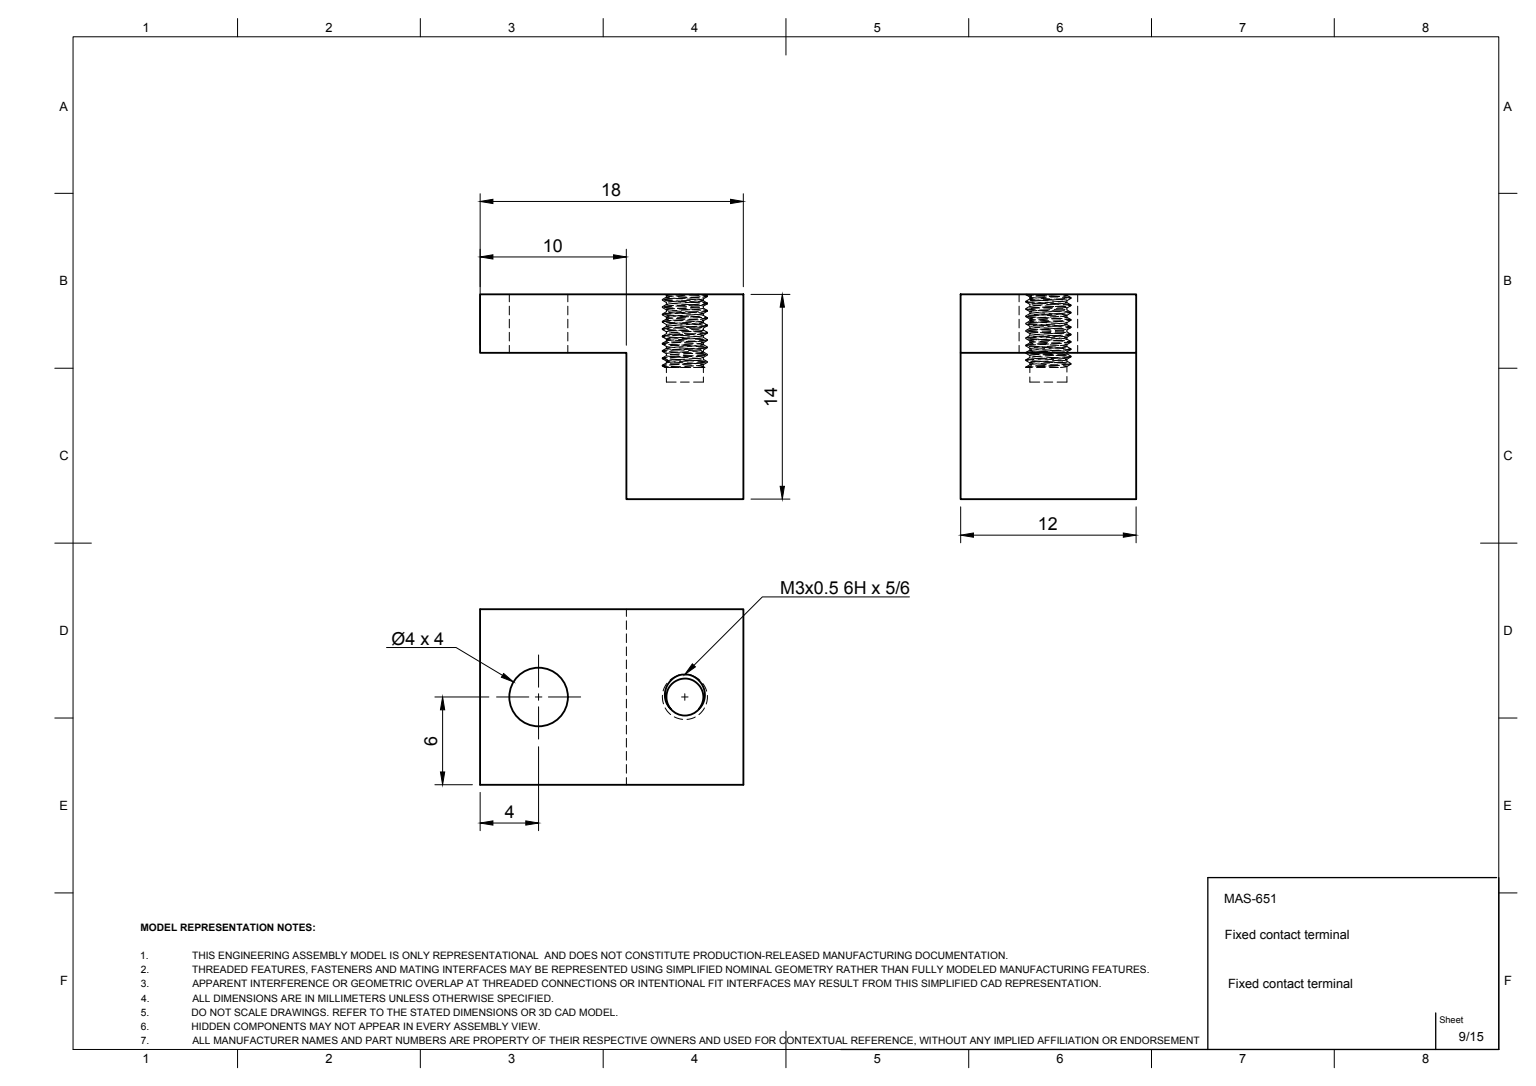
ISO-10303-21;
HEADER;
/* Generated by software containing ST-Developer
 * from STEP Tools, Inc. (www.steptools.com) 
 */

FILE_DESCRIPTION(
/* description */ ('Independent direct-acting normally-closed roller-plunger limit-switch
 CAD. Removable cover, insulated terminal supports, captured bus/conta
ct bridge, native Coil return spring, integral lower travel stop, reus
able instanced hardware and free roller. Manual geometric contact open
ing4mm; no snap-action/contact-force, electrical/current/voltage, envi
ronmental seal, safety-switch, wear, load or life certification. Exter
nal wiring and anchors omitted; fits and application engineering requi
red.'),
/* implementation_level */ '2;1');

FILE_NAME(
/* name */ 'Fixed contact terminal.step',
/* time_stamp */ '2026-11-08T07:32:43-08:00',
/* author */ (''),
/* organization */ (''),
/* preprocessor_version */ 'ST-DEVELOPER v20.2',
/* originating_system */ 'Autodesk Translation Framework v15.17.0.0',
/* authorisation */ '');

FILE_SCHEMA (('AUTOMOTIVE_DESIGN { 1 0 10303 214 3 1 1 }'));
ENDSEC;

DATA;
#10=MECHANICAL_DESIGN_GEOMETRIC_PRESENTATION_REPRESENTATION('',(#183),#36482);
#149=SHAPE_REPRESENTATION_RELATIONSHIP('SRR','None',#36562,#166);
#166=ADVANCED_BREP_SHAPE_REPRESENTATION('',(#200),#36472);
#183=STYLED_ITEM('',(#36653),#200);
#200=MANIFOLD_SOLID_BREP('Body1',#9774);
#226=B_SPLINE_SURFACE_WITH_KNOTS('',3,3,((#28474,#28475,#28476,#28477,#28478,
#28479,#28480,#28481,#28482,#28483,#28484,#28485,#28486,#28487,#28488,#28489,
#28490,#28491,#28492,#28493,#28494,#28495,#28496,#28497,#28498,#28499,#28500,
#28501,#28502,#28503,#28504,#28505,#28506,#28507,#28508,#28509,#28510,#28511,
#28512,#28513,#28514,#28515,#28516,#28517,#28518,#28519,#28520,#28521,#28522,
#28523,#28524,#28525,#28526,#28527,#28528,#28529,#28530,#28531,#28532,#28533,
#28534,#28535,#28536,#28537,#28538,#28539,#28540,#28541),(#28542,#28543,
#28544,#28545,#28546,#28547,#28548,#28549,#28550,#28551,#28552,#28553,#28554,
#28555,#28556,#28557,#28558,#28559,#28560,#28561,#28562,#28563,#28564,#28565,
#28566,#28567,#28568,#28569,#28570,#28571,#28572,#28573,#28574,#28575,#28576,
#28577,#28578,#28579,#28580,#28581,#28582,#28583,#28584,#28585,#28586,#28587,
#28588,#28589,#28590,#28591,#28592,#28593,#28594,#28595,#28596,#28597,#28598,
#28599,#28600,#28601,#28602,#28603,#28604,#28605,#28606,#28607,#28608,#28609),
(#28610,#28611,#28612,#28613,#28614,#28615,#28616,#28617,#28618,#28619,
#28620,#28621,#28622,#28623,#28624,#28625,#28626,#28627,#28628,#28629,#28630,
#28631,#28632,#28633,#28634,#28635,#28636,#28637,#28638,#28639,#28640,#28641,
#28642,#28643,#28644,#28645,#28646,#28647,#28648,#28649,#28650,#28651,#28652,
#28653,#28654,#28655,#28656,#28657,#28658,#28659,#28660,#28661,#28662,#28663,
#28664,#28665,#28666,#28667,#28668,#28669,#28670,#28671,#28672,#28673,#28674,
#28675,#28676,#28677),(#28678,#28679,#28680,#28681,#28682,#28683,#28684,
#28685,#28686,#28687,#28688,#28689,#28690,#28691,#28692,#28693,#28694,#28695,
#28696,#28697,#28698,#28699,#28700,#28701,#28702,#28703,#28704,#28705,#28706,
#28707,#28708,#28709,#28710,#28711,#28712,#28713,#28714,#28715,#28716,#28717,
#28718,#28719,#28720,#28721,#28722,#28723,#28724,#28725,#28726,#28727,#28728,
#28729,#28730,#28731,#28732,#28733,#28734,#28735,#28736,#28737,#28738,#28739,
#28740,#28741,#28742,#28743,#28744,#28745)),.UNSPECIFIED.,.F.,.F.,.F.,(4,
4),(4,1,1,1,1,1,1,1,1,1,1,1,1,1,1,1,1,1,1,1,1,1,1,1,1,1,1,1,1,1,1,1,1,1,
1,1,1,1,1,1,1,1,1,1,1,1,1,1,1,1,1,1,1,1,1,1,1,1,1,1,1,1,1,1,1,4),(0.,0.0321584099938621),
(11.8553612635792,12.8530908876339,13.8508205116886,14.8485501357432,15.8462797597979,
16.8440093838525,17.8417390079072,18.8394686319618,19.8371982560165,20.8349278800712,
21.8326575041258,22.8303871281805,23.8281167522351,24.8258463762898,25.8235760003445,
26.8213056243991,27.8190352484538,28.8167648725084,29.8144944965631,30.8122241206177,
31.8099537446724,32.8076833687271,33.8054129927817,34.8031426168364,35.800872240891,
36.7986018649457,37.7963314890004,38.794061113055,39.7917907371097,40.7895203611643,
41.787249985219,42.7849796092736,43.7827092333283,44.780438857383,45.7781684814376,
46.7758981054923,47.7736277295469,48.7713573536016,49.7690869776563,50.7668166017109,
51.7645462257656,52.7622758498202,53.7600054738749,54.7577350979295,55.7554647219842,
56.7531943460389,57.7509239700935,58.7486535941482,59.7463832182028,60.7441128422575,
61.7418424663121,62.7395720903668,63.7373017144215,64.7350313384761,65.7327609625308,
66.7304905865854,67.7282202106401,68.7259498346948,69.7236794587494,70.7214090828041,
71.7191387068587,72.7168683309134,73.7145979549681,74.7123275790227,75.7100572030774,
76.707786827132),.UNSPECIFIED.);
#227=B_SPLINE_SURFACE_WITH_KNOTS('',3,3,((#28820,#28821,#28822,#28823,#28824,
#28825,#28826,#28827,#28828,#28829,#28830,#28831,#28832,#28833,#28834,#28835,
#28836,#28837,#28838,#28839,#28840,#28841,#28842,#28843,#28844,#28845,#28846,
#28847,#28848,#28849,#28850,#28851,#28852,#28853,#28854,#28855,#28856,#28857,
#28858,#28859,#28860,#28861,#28862,#28863,#28864,#28865,#28866,#28867,#28868,
#28869,#28870,#28871,#28872,#28873,#28874,#28875,#28876,#28877,#28878,#28879,
#28880,#28881,#28882,#28883,#28884,#28885,#28886,#28887),(#28888,#28889,
#28890,#28891,#28892,#28893,#28894,#28895,#28896,#28897,#28898,#28899,#28900,
#28901,#28902,#28903,#28904,#28905,#28906,#28907,#28908,#28909,#28910,#28911,
#28912,#28913,#28914,#28915,#28916,#28917,#28918,#28919,#28920,#28921,#28922,
#28923,#28924,#28925,#28926,#28927,#28928,#28929,#28930,#28931,#28932,#28933,
#28934,#28935,#28936,#28937,#28938,#28939,#28940,#28941,#28942,#28943,#28944,
#28945,#28946,#28947,#28948,#28949,#28950,#28951,#28952,#28953,#28954,#28955),
(#28956,#28957,#28958,#28959,#28960,#28961,#28962,#28963,#28964,#28965,
#28966,#28967,#28968,#28969,#28970,#28971,#28972,#28973,#28974,#28975,#28976,
#28977,#28978,#28979,#28980,#28981,#28982,#28983,#28984,#28985,#28986,#28987,
#28988,#28989,#28990,#28991,#28992,#28993,#28994,#28995,#28996,#28997,#28998,
#28999,#29000,#29001,#29002,#29003,#29004,#29005,#29006,#29007,#29008,#29009,
#29010,#29011,#29012,#29013,#29014,#29015,#29016,#29017,#29018,#29019,#29020,
#29021,#29022,#29023),(#29024,#29025,#29026,#29027,#29028,#29029,#29030,
#29031,#29032,#29033,#29034,#29035,#29036,#29037,#29038,#29039,#29040,#29041,
#29042,#29043,#29044,#29045,#29046,#29047,#29048,#29049,#29050,#29051,#29052,
#29053,#29054,#29055,#29056,#29057,#29058,#29059,#29060,#29061,#29062,#29063,
#29064,#29065,#29066,#29067,#29068,#29069,#29070,#29071,#29072,#29073,#29074,
#29075,#29076,#29077,#29078,#29079,#29080,#29081,#29082,#29083,#29084,#29085,
#29086,#29087,#29088,#29089,#29090,#29091)),.UNSPECIFIED.,.F.,.F.,.F.,(4,
4),(4,1,1,1,1,1,1,1,1,1,1,1,1,1,1,1,1,1,1,1,1,1,1,1,1,1,1,1,1,1,1,1,1,1,
1,1,1,1,1,1,1,1,1,1,1,1,1,1,1,1,1,1,1,1,1,1,1,1,1,1,1,1,1,1,1,4),(0.,0.0321584099938616),
(14.3984001269718,15.3961297510265,16.3938593750811,17.3915889991358,18.3893186231905,
19.3870482472451,20.3847778712998,21.3825074953544,22.3802371194091,23.3779667434637,
24.3756963675184,25.3734259915731,26.3711556156277,27.3688852396824,28.366614863737,
29.3643444877917,30.3620741118463,31.359803735901,32.3575333599556,33.3552629840103,
34.352992608065,35.3507222321196,36.3484518561743,37.3461814802289,38.3439111042836,
39.3416407283382,40.3393703523929,41.3370999764475,42.3348296005022,43.3325592245569,
44.3302888486115,45.3280184726662,46.3257480967208,47.3234777207755,48.3212073448301,
49.3189369688848,50.3166665929395,51.3143962169941,52.3121258410488,53.3098554651034,
54.3075850891581,55.3053147132127,56.3030443372674,57.3007739613221,58.2985035853767,
59.2962332094314,60.293962833486,61.2916924575407,62.2894220815953,63.28715170565,
64.2848813297046,65.2826109537593,66.280340577814,67.2780702018686,68.2757998259233,
69.2735294499779,70.2712590740326,71.2689886980872,72.2667183221419,73.2644479461966,
74.2621775702512,75.2599071943059,76.2576368183605,77.2553664424152,78.2530960664698,
79.2508256905245),.UNSPECIFIED.);
#284=FACE_BOUND('',#1389,.T.);
#285=FACE_BOUND('',#1395,.T.);
#286=FACE_BOUND('',#1396,.T.);
#378=PLANE('',#10428);
#379=PLANE('',#10431);
#380=PLANE('',#10435);
#381=PLANE('',#10436);
#382=PLANE('',#10437);
#383=PLANE('',#10438);
#384=PLANE('',#10439);
#385=PLANE('',#10440);
#386=PLANE('',#10441);
#387=PLANE('',#10442);
#773=FACE_OUTER_BOUND('',#1360,.T.);
#774=FACE_OUTER_BOUND('',#1361,.T.);
#775=FACE_OUTER_BOUND('',#1362,.T.);
#776=FACE_OUTER_BOUND('',#1363,.T.);
#777=FACE_OUTER_BOUND('',#1364,.T.);
#778=FACE_OUTER_BOUND('',#1365,.T.);
#779=FACE_OUTER_BOUND('',#1366,.T.);
#780=FACE_OUTER_BOUND('',#1367,.T.);
#781=FACE_OUTER_BOUND('',#1368,.T.);
#782=FACE_OUTER_BOUND('',#1369,.T.);
#783=FACE_OUTER_BOUND('',#1370,.T.);
#784=FACE_OUTER_BOUND('',#1371,.T.);
#785=FACE_OUTER_BOUND('',#1372,.T.);
#786=FACE_OUTER_BOUND('',#1373,.T.);
#787=FACE_OUTER_BOUND('',#1374,.T.);
#788=FACE_OUTER_BOUND('',#1375,.T.);
#789=FACE_OUTER_BOUND('',#1376,.T.);
#790=FACE_OUTER_BOUND('',#1377,.T.);
#791=FACE_OUTER_BOUND('',#1378,.T.);
#792=FACE_OUTER_BOUND('',#1379,.T.);
#793=FACE_OUTER_BOUND('',#1380,.T.);
#794=FACE_OUTER_BOUND('',#1381,.T.);
#795=FACE_OUTER_BOUND('',#1382,.T.);
#796=FACE_OUTER_BOUND('',#1383,.T.);
#797=FACE_OUTER_BOUND('',#1384,.T.);
#798=FACE_OUTER_BOUND('',#1385,.T.);
#799=FACE_OUTER_BOUND('',#1386,.T.);
#800=FACE_OUTER_BOUND('',#1387,.T.);
#801=FACE_OUTER_BOUND('',#1388,.T.);
#802=FACE_OUTER_BOUND('',#1390,.T.);
#803=FACE_OUTER_BOUND('',#1391,.T.);
#804=FACE_OUTER_BOUND('',#1392,.T.);
#805=FACE_OUTER_BOUND('',#1393,.T.);
#806=FACE_OUTER_BOUND('',#1394,.T.);
#807=FACE_OUTER_BOUND('',#1397,.T.);
#1360=EDGE_LOOP('',(#7816,#7817,#7818,#7819,#7820,#7821,#7822,#7823));
#1361=EDGE_LOOP('',(#7824,#7825,#7826,#7827));
#1362=EDGE_LOOP('',(#7828,#7829,#7830,#7831));
#1363=EDGE_LOOP('',(#7832,#7833,#7834,#7835));
#1364=EDGE_LOOP('',(#7836,#7837,#7838,#7839));
#1365=EDGE_LOOP('',(#7840,#7841,#7842,#7843));
#1366=EDGE_LOOP('',(#7844,#7845,#7846,#7847));
#1367=EDGE_LOOP('',(#7848,#7849,#7850,#7851));
#1368=EDGE_LOOP('',(#7852,#7853,#7854,#7855));
#1369=EDGE_LOOP('',(#7856,#7857,#7858,#7859));
#1370=EDGE_LOOP('',(#7860,#7861,#7862,#7863));
#1371=EDGE_LOOP('',(#7864,#7865,#7866,#7867));
#1372=EDGE_LOOP('',(#7868,#7869,#7870,#7871));
#1373=EDGE_LOOP('',(#7872,#7873,#7874,#7875));
#1374=EDGE_LOOP('',(#7876,#7877,#7878,#7879));
#1375=EDGE_LOOP('',(#7880,#7881,#7882,#7883));
#1376=EDGE_LOOP('',(#7884,#7885,#7886,#7887));
#1377=EDGE_LOOP('',(#7888,#7889,#7890,#7891));
#1378=EDGE_LOOP('',(#7892,#7893,#7894,#7895));
#1379=EDGE_LOOP('',(#7896,#7897,#7898,#7899));
#1380=EDGE_LOOP('',(#7900,#7901,#7902,#7903,#7904));
#1381=EDGE_LOOP('',(#7905,#7906,#7907,#7908));
#1382=EDGE_LOOP('',(#7909,#7910,#7911,#7912,#7913,#7914,#7915,#7916,#7917,
#7918,#7919,#7920,#7921,#7922,#7923,#7924,#7925,#7926,#7927,#7928,#7929,
#7930,#7931,#7932));
#1383=EDGE_LOOP('',(#7933,#7934,#7935,#7936,#7937,#7938,#7939,#7940,#7941,
#7942,#7943,#7944,#7945,#7946,#7947,#7948,#7949,#7950,#7951,#7952,#7953,
#7954,#7955,#7956));
#1384=EDGE_LOOP('',(#7957,#7958,#7959,#7960));
#1385=EDGE_LOOP('',(#7961));
#1386=EDGE_LOOP('',(#7962,#7963,#7964,#7965));
#1387=EDGE_LOOP('',(#7966,#7967,#7968,#7969));
#1388=EDGE_LOOP('',(#7970,#7971,#7972,#7973));
#1389=EDGE_LOOP('',(#7974));
#1390=EDGE_LOOP('',(#7975,#7976,#7977,#7978,#7979,#7980));
#1391=EDGE_LOOP('',(#7981,#7982,#7983,#7984));
#1392=EDGE_LOOP('',(#7985,#7986,#7987,#7988,#7989,#7990));
#1393=EDGE_LOOP('',(#7991,#7992,#7993,#7994));
#1394=EDGE_LOOP('',(#7995,#7996,#7997,#7998));
#1395=EDGE_LOOP('',(#7999,#8000,#8001,#8002));
#1396=EDGE_LOOP('',(#8003));
#1397=EDGE_LOOP('',(#8004,#8005,#8006,#8007));
#1685=CIRCLE('',#10403,0.12645);
#1686=CIRCLE('',#10404,0.12645);
#1687=CIRCLE('',#10405,0.12645);
#1688=CIRCLE('',#10415,0.12645);
#1689=CIRCLE('',#10417,0.1543);
#1690=CIRCLE('',#10427,0.1543);
#1691=CIRCLE('',#10433,0.2);
#1692=CIRCLE('',#10434,0.2);
#2193=B_SPLINE_CURVE_WITH_KNOTS('',3,(#27648,#27649,#27650,#27651),
 .UNSPECIFIED.,.F.,.F.,(4,4),(64.1414162127729,64.8524255635527),
 .UNSPECIFIED.);
#2194=B_SPLINE_CURVE_WITH_KNOTS('',3,(#27659,#27660,#27661,#27662,#27663,
#27664,#27665,#27666,#27667,#27668),.UNSPECIFIED.,.F.,.F.,(4,3,3,4),(-62.8318530717959,
-61.8592366913888,-60.8615070673342,-60.401269768986),.UNSPECIFIED.);
#2195=B_SPLINE_CURVE_WITH_KNOTS('',3,(#27673,#27674,#27675,#27676,#27677,
#27678,#27679,#27680,#27681,#27682,#27683,#27684,#27685,#27686,#27687,#27688,
#27689,#27690,#27691,#27692,#27693,#27694,#27695,#27696,#27697),
 .UNSPECIFIED.,.F.,.F.,(4,3,3,3,3,3,3,3,4),(57.8582309055934,57.8683181951701,
58.8660478192247,59.8637774432794,60.861507067334,61.8592366913887,62.8569663154434,
63.854695939498,64.1414162127729),.UNSPECIFIED.);
#2196=B_SPLINE_CURVE_WITH_KNOTS('',3,(#27698,#27699,#27700,#27701,#27702,
#27703,#27704,#27705,#27706,#27707,#27708,#27709,#27710,#27711,#27712,#27713,
#27714,#27715,#27716,#27717,#27718,#27719),.UNSPECIFIED.,.F.,.F.,(4,3,3,
3,3,3,3,4),(-60.401269768986,-59.8637774432795,-58.8660478192248,-57.8683181951702,
-56.8705885711155,-55.8728589470609,-54.8751293230062,-54.1180844618064),
 .UNSPECIFIED.);
#2197=B_SPLINE_CURVE_WITH_KNOTS('',3,(#27724,#27725,#27726,#27727,#27728,
#27729,#27730,#27731,#27732,#27733,#27734,#27735,#27736,#27737,#27738,#27739,
#27740,#27741,#27742,#27743,#27744,#27745),.UNSPECIFIED.,.F.,.F.,(4,3,3,
3,3,3,3,4),(51.5750455984138,51.8819404508421,52.8796700748968,53.8773996989514,
54.8751293230061,55.8728589470608,56.8705885711154,57.8582309055934),
 .UNSPECIFIED.);
#2198=B_SPLINE_CURVE_WITH_KNOTS('',3,(#27746,#27747,#27748,#27749,#27750,
#27751,#27752,#27753,#27754,#27755,#27756,#27757,#27758,#27759,#27760,#27761,
#27762,#27763,#27764,#27765,#27766,#27767,#27768,#27769,#27770),
 .UNSPECIFIED.,.F.,.F.,(4,3,3,3,3,3,3,3,4),(-54.1180844618064,-53.8773996989516,
-52.8796700748969,-51.8819404508422,-50.8842108267876,-49.8864812027329,
-48.8887515786783,-47.8910219546236,-47.8348991546268),.UNSPECIFIED.);
#2199=B_SPLINE_CURVE_WITH_KNOTS('',3,(#27775,#27776,#27777,#27778,#27779,
#27780,#27781,#27782,#27783,#27784,#27785,#27786,#27787,#27788,#27789,#27790,
#27791,#27792,#27793,#27794,#27795,#27796),.UNSPECIFIED.,.F.,.F.,(4,3,3,
3,3,3,3,4),(45.2918602912342,45.8955627065142,46.8932923305688,47.8910219546235,
48.8887515786782,49.8864812027328,50.8842108267875,51.5750455984138),
 .UNSPECIFIED.);
#2200=B_SPLINE_CURVE_WITH_KNOTS('',3,(#27797,#27798,#27799,#27800,#27801,
#27802,#27803,#27804,#27805,#27806,#27807,#27808,#27809,#27810,#27811,#27812,
#27813,#27814,#27815,#27816,#27817,#27818),.UNSPECIFIED.,.F.,.F.,(4,3,3,
3,3,3,3,4),(-47.8348991546268,-46.8932923305689,-45.8955627065143,-44.8978330824596,
-43.900103458405,-42.9023738343503,-41.9046442102957,-41.5517138474472),
 .UNSPECIFIED.);
#2201=B_SPLINE_CURVE_WITH_KNOTS('',3,(#27823,#27824,#27825,#27826,#27827,
#27828,#27829,#27830,#27831,#27832,#27833,#27834,#27835,#27836,#27837,#27838,
#27839,#27840,#27841,#27842,#27843,#27844),.UNSPECIFIED.,.F.,.F.,(4,3,3,
3,3,3,3,4),(39.0086749840546,39.9091849621863,40.9069145862409,41.9046442102956,
42.9023738343502,43.9001034584049,44.8978330824595,45.2918602912342),
 .UNSPECIFIED.);
#2202=B_SPLINE_CURVE_WITH_KNOTS('',3,(#27845,#27846,#27847,#27848,#27849,
#27850,#27851,#27852,#27853,#27854,#27855,#27856,#27857,#27858,#27859,#27860,
#27861,#27862,#27863,#27864,#27865,#27866),.UNSPECIFIED.,.F.,.F.,(4,3,3,
3,3,3,3,4),(-41.5517138474472,-40.906914586241,-39.9091849621863,-38.9114553381317,
-37.913725714077,-36.9159960900224,-35.9182664659677,-35.2685285402676),
 .UNSPECIFIED.);
#2203=B_SPLINE_CURVE_WITH_KNOTS('',3,(#27871,#27872,#27873,#27874,#27875,
#27876,#27877,#27878,#27879,#27880,#27881,#27882,#27883,#27884,#27885,#27886,
#27887,#27888,#27889,#27890,#27891,#27892,#27893,#27894,#27895),
 .UNSPECIFIED.,.F.,.F.,(4,3,3,3,3,3,3,3,4),(32.725489676875,32.9250775938037,
33.9228072178583,34.920536841913,35.9182664659676,36.9159960900223,37.9137257140769,
38.9114553381316,39.0086749840546),.UNSPECIFIED.);
#2204=B_SPLINE_CURVE_WITH_KNOTS('',3,(#27896,#27897,#27898,#27899,#27900,
#27901,#27902,#27903,#27904,#27905,#27906,#27907,#27908,#27909,#27910,#27911,
#27912,#27913,#27914,#27915,#27916,#27917),.UNSPECIFIED.,.F.,.F.,(4,3,3,
3,3,3,3,4),(-35.2685285402676,-34.920536841913,-33.9228072178584,-32.9250775938037,
-31.9273479697491,-30.9296183456944,-29.9318887216397,-28.985343233088),
 .UNSPECIFIED.);
#2205=B_SPLINE_CURVE_WITH_KNOTS('',3,(#27922,#27923,#27924,#27925,#27926,
#27927,#27928,#27929,#27930,#27931,#27932,#27933,#27934,#27935,#27936,#27937,
#27938,#27939,#27940,#27941,#27942,#27943),.UNSPECIFIED.,.F.,.F.,(4,3,3,
3,3,3,3,4),(26.4423043696954,26.9386998494757,27.9364294735304,28.934159097585,
29.9318887216397,30.9296183456943,31.927347969749,32.725489676875),
 .UNSPECIFIED.);
#2206=B_SPLINE_CURVE_WITH_KNOTS('',3,(#27944,#27945,#27946,#27947,#27948,
#27949,#27950,#27951,#27952,#27953,#27954,#27955,#27956,#27957,#27958,#27959,
#27960,#27961,#27962,#27963,#27964,#27965,#27966,#27967,#27968),
 .UNSPECIFIED.,.F.,.F.,(4,3,3,3,3,3,3,3,4),(-28.985343233088,-28.9341590975851,
-27.9364294735304,-26.9386998494758,-25.9409702254211,-24.9432406013665,
-23.9455109773118,-22.9477813532571,-22.7021579259084),.UNSPECIFIED.);
#2207=B_SPLINE_CURVE_WITH_KNOTS('',3,(#27973,#27974,#27975,#27976,#27977,
#27978,#27979,#27980,#27981,#27982,#27983,#27984,#27985,#27986,#27987,#27988,
#27989,#27990,#27991,#27992,#27993,#27994),.UNSPECIFIED.,.F.,.F.,(4,3,3,
3,3,3,3,4),(20.1591190625158,20.9523221051478,21.9500517292024,22.9477813532571,
23.9455109773117,24.9432406013664,25.9409702254211,26.4423043696954),
 .UNSPECIFIED.);
#2208=B_SPLINE_CURVE_WITH_KNOTS('',3,(#27995,#27996,#27997,#27998,#27999,
#28000,#28001,#28002,#28003,#28004,#28005,#28006,#28007,#28008,#28009,#28010,
#28011,#28012,#28013,#28014,#28015,#28016),.UNSPECIFIED.,.F.,.F.,(4,3,3,
3,3,3,3,4),(-22.7021579259084,-21.9500517292025,-20.9523221051478,-19.9545924810932,
-18.9568628570385,-17.9591332329838,-16.9614036089292,-16.4189726187288),
 .UNSPECIFIED.);
#2209=B_SPLINE_CURVE_WITH_KNOTS('',3,(#28021,#28022,#28023,#28024,#28025,
#28026,#28027,#28028,#28029,#28030,#28031,#28032,#28033,#28034,#28035,#28036,
#28037,#28038,#28039,#28040,#28041,#28042,#28043,#28044,#28045),
 .UNSPECIFIED.,.F.,.F.,(4,3,3,3,3,3,3,3,4),(13.8759337553362,13.9682147367652,
14.9659443608198,15.9636739848745,16.9614036089292,17.9591332329838,18.9568628570385,
19.9545924810931,20.1591190625158),.UNSPECIFIED.);
#2210=B_SPLINE_CURVE_WITH_KNOTS('',3,(#28046,#28047,#28048,#28049,#28050,
#28051,#28052,#28053,#28054,#28055,#28056,#28057,#28058,#28059,#28060,#28061,
#28062,#28063,#28064,#28065,#28066,#28067),.UNSPECIFIED.,.F.,.F.,(4,3,3,
3,3,3,3,4),(-16.4189726187288,-15.9636739848745,-14.9659443608199,-13.9682147367652,
-12.9704851127106,-11.9727554886559,-10.9750258646012,-10.1357873115493),
 .UNSPECIFIED.);
#2211=B_SPLINE_CURVE_WITH_KNOTS('',3,(#28073,#28074,#28075,#28076,#28077,
#28078,#28079,#28080,#28081,#28082,#28083,#28084,#28085),.UNSPECIFIED.,
 .F.,.F.,(4,3,3,3,4),(-3.85260200436966,-2.99318887216398,-1.99545924810932,
-0.997729624054659,0.),.UNSPECIFIED.);
#2212=B_SPLINE_CURVE_WITH_KNOTS('',3,(#28088,#28089,#28090,#28091,#28092,
#28093,#28094,#28095,#28096,#28097,#28098,#28099,#28100,#28101,#28102,#28103,
#28104,#28105,#28106),.UNSPECIFIED.,.F.,.F.,(4,3,3,3,3,3,4),(2.02057249175679,
2.99318887216397,3.99091849621862,4.98864812027328,5.98637774432793,6.98410736838259,
7.59274844815664),.UNSPECIFIED.);
#2213=B_SPLINE_CURVE_WITH_KNOTS('',3,(#28112,#28113,#28114,#28115,#28116,
#28117,#28118,#28119),.UNSPECIFIED.,.F.,.F.,(4,1,1,1,1,4),(72.2566310325653,
72.7168683309134,73.7145979549681,74.7123275790227,75.7100572030774,76.707786827132),
 .UNSPECIFIED.);
#2214=B_SPLINE_CURVE_WITH_KNOTS('',3,(#28122,#28123,#28124,#28125,#28126,
#28127,#28128,#28129,#28130),.UNSPECIFIED.,.F.,.F.,(4,1,1,1,1,1,4),(72.2566310325653,
72.2667183221419,73.2644479461966,74.2621775702512,75.2599071943059,76.2576368183605,
77.2302531987677),.UNSPECIFIED.);
#2215=B_SPLINE_CURVE_WITH_KNOTS('',3,(#28135,#28136,#28137,#28138,#28139,
#28140,#28141,#28142,#28143,#28144),.UNSPECIFIED.,.F.,.F.,(4,1,1,1,1,1,
1,4),(65.9734457253856,66.7304905865854,67.7282202106401,68.7259498346948,
69.7236794587494,70.7214090828041,71.7191387068587,72.2566310325653),
 .UNSPECIFIED.);
#2216=B_SPLINE_CURVE_WITH_KNOTS('',3,(#28145,#28146,#28147,#28148,#28149,
#28150,#28151,#28152,#28153,#28154),.UNSPECIFIED.,.F.,.F.,(4,1,1,1,1,1,
1,4),(65.9734457253856,66.280340577814,67.2780702018686,68.2757998259233,
69.2735294499779,70.2712590740326,71.2689886980872,72.2566310325653),
 .UNSPECIFIED.);
#2217=B_SPLINE_CURVE_WITH_KNOTS('',3,(#28159,#28160,#28161,#28162,#28163,
#28164,#28165,#28166,#28167,#28168,#28169),.UNSPECIFIED.,.F.,.F.,(4,1,1,
1,1,1,1,1,4),(59.690260418206,59.7463832182028,60.7441128422575,61.7418424663121,
62.7395720903668,63.7373017144215,64.7350313384761,65.7327609625308,65.9734457253856),
 .UNSPECIFIED.);
#2218=B_SPLINE_CURVE_WITH_KNOTS('',3,(#28170,#28171,#28172,#28173,#28174,
#28175,#28176,#28177,#28178,#28179),.UNSPECIFIED.,.F.,.F.,(4,1,1,1,1,1,
1,4),(59.690260418206,60.293962833486,61.2916924575407,62.2894220815953,
63.28715170565,64.2848813297046,65.2826109537593,65.9734457253856),
 .UNSPECIFIED.);
#2219=B_SPLINE_CURVE_WITH_KNOTS('',3,(#28184,#28185,#28186,#28187,#28188,
#28189,#28190,#28191,#28192,#28193),.UNSPECIFIED.,.F.,.F.,(4,1,1,1,1,1,
1,4),(53.4070751110265,53.7600054738749,54.7577350979295,55.7554647219842,
56.7531943460389,57.7509239700935,58.7486535941482,59.690260418206),
 .UNSPECIFIED.);
#2220=B_SPLINE_CURVE_WITH_KNOTS('',3,(#28194,#28195,#28196,#28197,#28198,
#28199,#28200,#28201,#28202,#28203),.UNSPECIFIED.,.F.,.F.,(4,1,1,1,1,1,
1,4),(53.4070751110265,54.3075850891581,55.3053147132127,56.3030443372674,
57.3007739613221,58.2985035853767,59.2962332094314,59.690260418206),
 .UNSPECIFIED.);
#2221=B_SPLINE_CURVE_WITH_KNOTS('',3,(#28208,#28209,#28210,#28211,#28212,
#28213,#28214,#28215,#28216,#28217),.UNSPECIFIED.,.F.,.F.,(4,1,1,1,1,1,
1,4),(47.1238898038468,47.7736277295469,48.7713573536016,49.7690869776563,
50.7668166017109,51.7645462257656,52.7622758498202,53.4070751110265),
 .UNSPECIFIED.);
#2222=B_SPLINE_CURVE_WITH_KNOTS('',3,(#28218,#28219,#28220,#28221,#28222,
#28223,#28224,#28225,#28226,#28227,#28228),.UNSPECIFIED.,.F.,.F.,(4,1,1,
1,1,1,1,1,4),(47.1238898038468,47.3234777207755,48.3212073448301,49.3189369688848,
50.3166665929395,51.3143962169941,52.3121258410488,53.3098554651034,53.4070751110265),
 .UNSPECIFIED.);
#2223=B_SPLINE_CURVE_WITH_KNOTS('',3,(#28233,#28234,#28235,#28236,#28237,
#28238,#28239,#28240,#28241,#28242),.UNSPECIFIED.,.F.,.F.,(4,1,1,1,1,1,
1,4),(40.8407044966673,41.787249985219,42.7849796092736,43.7827092333283,
44.780438857383,45.7781684814376,46.7758981054923,47.1238898038468),
 .UNSPECIFIED.);
#2224=B_SPLINE_CURVE_WITH_KNOTS('',3,(#28243,#28244,#28245,#28246,#28247,
#28248,#28249,#28250,#28251,#28252),.UNSPECIFIED.,.F.,.F.,(4,1,1,1,1,1,
1,4),(40.8407044966673,41.3370999764475,42.3348296005022,43.3325592245569,
44.3302888486115,45.3280184726662,46.3257480967208,47.1238898038468),
 .UNSPECIFIED.);
#2225=B_SPLINE_CURVE_WITH_KNOTS('',3,(#28257,#28258,#28259,#28260,#28261,
#28262,#28263,#28264,#28265,#28266,#28267),.UNSPECIFIED.,.F.,.F.,(4,1,1,
1,1,1,1,1,4),(34.5575191894877,34.8031426168364,35.800872240891,36.7986018649457,
37.7963314890004,38.794061113055,39.7917907371097,40.7895203611643,40.8407044966673),
 .UNSPECIFIED.);
#2226=B_SPLINE_CURVE_WITH_KNOTS('',3,(#28268,#28269,#28270,#28271,#28272,
#28273,#28274,#28275,#28276,#28277),.UNSPECIFIED.,.F.,.F.,(4,1,1,1,1,1,
1,4),(34.5575191894877,35.3507222321196,36.3484518561743,37.3461814802289,
38.3439111042836,39.3416407283382,40.3393703523929,40.8407044966673),
 .UNSPECIFIED.);
#2227=B_SPLINE_CURVE_WITH_KNOTS('',3,(#28282,#28283,#28284,#28285,#28286,
#28287,#28288,#28289,#28290,#28291),.UNSPECIFIED.,.F.,.F.,(4,1,1,1,1,1,
1,4),(28.2743338823081,28.8167648725084,29.8144944965631,30.8122241206177,
31.8099537446724,32.8076833687271,33.8054129927817,34.5575191894877),
 .UNSPECIFIED.);
#2228=B_SPLINE_CURVE_WITH_KNOTS('',3,(#28292,#28293,#28294,#28295,#28296,
#28297,#28298,#28299,#28300,#28301,#28302),.UNSPECIFIED.,.F.,.F.,(4,1,1,
1,1,1,1,1,4),(28.2743338823081,28.366614863737,29.3643444877917,30.3620741118463,
31.359803735901,32.3575333599556,33.3552629840103,34.352992608065,34.5575191894877),
 .UNSPECIFIED.);
#2229=B_SPLINE_CURVE_WITH_KNOTS('',3,(#28307,#28308,#28309,#28310,#28311,
#28312,#28313,#28314,#28315,#28316),.UNSPECIFIED.,.F.,.F.,(4,1,1,1,1,1,
1,4),(21.9911485751285,22.8303871281805,23.8281167522351,24.8258463762898,
25.8235760003445,26.8213056243991,27.8190352484538,28.2743338823081),
 .UNSPECIFIED.);
#2230=B_SPLINE_CURVE_WITH_KNOTS('',3,(#28317,#28318,#28319,#28320,#28321,
#28322,#28323,#28324,#28325,#28326),.UNSPECIFIED.,.F.,.F.,(4,1,1,1,1,1,
1,4),(21.9911485751285,22.3802371194091,23.3779667434637,24.3756963675184,
25.3734259915731,26.3711556156277,27.3688852396824,28.2743338823081),
 .UNSPECIFIED.);
#2231=B_SPLINE_CURVE_WITH_KNOTS('',3,(#28332,#28333,#28334,#28335,#28336),
 .UNSPECIFIED.,.F.,.F.,(4,1,4),(14.3984001269718,15.3961297510265,15.7079632679489),
 .UNSPECIFIED.);
#2232=B_SPLINE_CURVE_WITH_KNOTS('',3,(#28339,#28340,#28341,#28342,#28343),
 .UNSPECIFIED.,.F.,.F.,(4,1,4),(13.8759337553361,14.8485501357432,15.7079632679489),
 .UNSPECIFIED.);
#2233=B_SPLINE_CURVE_WITH_KNOTS('',3,(#28345,#28346,#28347,#28348,#28349,
#28350,#28351,#28352,#28353,#28354,#28355,#28356,#28357,#28358,#28359,#28360,
#28361,#28362,#28363,#28364,#28365,#28366,#28367,#28368,#28369,#28370,#28371,
#28372,#28373,#28374,#28375,#28376,#28377,#28378,#28379,#28380,#28381,#28382,
#28383,#28384,#28385,#28386,#28387,#28388,#28389,#28390,#28391,#28392,#28393,
#28394,#28395,#28396),.UNSPECIFIED.,.F.,.F.,(4,3,3,3,3,3,3,3,3,3,3,3,3,
3,3,3,3,4),(-0.286347380332243,-0.266225517657927,-0.253989633145399,-0.224118418951897,
-0.213637228539926,-0.18277997814213,-0.1712802294816,-0.161583702204544,
-0.151922727744335,-0.129977880386141,-0.117970426661857,-0.109303558462843,
-0.0829498108000933,-0.0663205445941391,-0.0521986510922473,-0.0198616494821571,
-0.00388856781184301,0.),.UNSPECIFIED.);
#2234=B_SPLINE_CURVE_WITH_KNOTS('',3,(#28397,#28398,#28399,#28400,#28401,
#28402,#28403,#28404,#28405,#28406,#28407,#28408,#28409,#28410,#28411,#28412,
#28413,#28414,#28415,#28416,#28417,#28418,#28419,#28420,#28421,#28422,#28423,
#28424,#28425,#28426,#28427,#28428,#28429,#28430,#28431,#28432,#28433,#28434,
#28435,#28436,#28437,#28438,#28439,#28440,#28441,#28442,#28443,#28444,#28445,
#28446,#28447,#28448,#28449,#28450,#28451),.UNSPECIFIED.,.F.,.F.,(4,3,3,
3,3,3,3,3,3,3,3,3,3,3,3,3,3,3,4),(-0.285142803995136,-0.264771978453909,
-0.248971203111392,-0.236527824899921,-0.214293390992849,-0.2038268270722,
-0.17295400685889,-0.159192875564253,-0.149652609754856,-0.137562774558619,
-0.11631964633286,-0.104925727456541,-0.0956925453293139,-0.0725695145406395,
-0.0586514835868502,-0.0490375298028169,-0.0212486353032901,-0.00320042217461625,
0.),.UNSPECIFIED.);
#2235=B_SPLINE_CURVE_WITH_KNOTS('',3,(#28453,#28454,#28455,#28456,#28457,
#28458,#28459,#28460,#28461,#28462,#28463),.UNSPECIFIED.,.F.,.F.,(4,1,1,
1,1,1,1,1,4),(15.7079632679489,15.8462797597979,16.8440093838525,17.8417390079072,
18.8394686319618,19.8371982560165,20.8349278800712,21.8326575041258,21.9911485751285),
 .UNSPECIFIED.);
#2236=B_SPLINE_CURVE_WITH_KNOTS('',3,(#28464,#28465,#28466,#28467,#28468,
#28469,#28470,#28471,#28472,#28473),.UNSPECIFIED.,.F.,.F.,(4,1,1,1,1,1,
1,4),(15.7079632679489,16.3938593750811,17.3915889991358,18.3893186231905,
19.3870482472451,20.3847778712998,21.3825074953544,21.9911485751285),
 .UNSPECIFIED.);
#2237=B_SPLINE_CURVE_WITH_KNOTS('',3,(#28746,#28747,#28748,#28749,#28750,
#28751,#28752,#28753,#28754,#28755,#28756,#28757,#28758,#28759,#28760,#28761,
#28762,#28763,#28764,#28765,#28766,#28767,#28768,#28769,#28770,#28771,#28772,
#28773,#28774,#28775,#28776,#28777,#28778,#28779,#28780,#28781,#28782,#28783,
#28784,#28785,#28786,#28787,#28788,#28789,#28790,#28791,#28792,#28793,#28794),
 .UNSPECIFIED.,.F.,.F.,(4,3,3,3,3,3,3,3,3,3,3,3,3,3,3,3,4),(0.,0.0274255371814078,
0.0484189866654049,0.0576777559231281,0.0872193790463039,0.100313119697051,
0.108749799500732,0.134012411342703,0.149997937188314,0.163168454336766,
0.192693763100972,0.210037636696566,0.220559059471184,0.247872294074534,
0.26049857837061,0.281269689393589,0.285142803995142),.UNSPECIFIED.);
#2238=B_SPLINE_CURVE_WITH_KNOTS('',3,(#28795,#28796,#28797,#28798,#28799,
#28800,#28801,#28802,#28803,#28804,#28805,#28806,#28807,#28808,#28809,#28810,
#28811,#28812,#28813,#28814,#28815,#28816,#28817,#28818,#28819),
 .UNSPECIFIED.,.F.,.F.,(4,3,3,3,3,3,3,3,4),(-10.1357873115493,-9.97729624054658,
-8.97956661649192,-7.98183699243727,-6.98410736838261,-5.98637774432795,
-4.98864812027329,-3.99091849621863,-3.85260200436966),.UNSPECIFIED.);
#2239=B_SPLINE_CURVE_WITH_KNOTS('',3,(#29092,#29093,#29094,#29095,#29096,
#29097,#29098,#29099,#29100,#29101,#29102,#29103,#29104,#29105,#29106,#29107,
#29108,#29109,#29110,#29111,#29112,#29113),.UNSPECIFIED.,.F.,.F.,(4,3,3,
3,3,3,3,4),(7.59274844815664,7.98183699243725,8.9795666164919,9.97729624054656,
10.9750258646012,11.9727554886559,12.9704851127105,13.8759337553362),
 .UNSPECIFIED.);
#2240=B_SPLINE_CURVE_WITH_KNOTS('',3,(#29114,#29115,#29116,#29117,#29118,
#29119,#29120,#29121,#29122,#29123,#29124,#29125,#29126,#29127,#29128,#29129,
#29130,#29131,#29132,#29133,#29134,#29135,#29136,#29137,#29138,#29139,#29140,
#29141,#29142,#29143,#29144,#29145,#29146,#29147,#29148,#29149,#29150,#29151,
#29152,#29153,#29154,#29155,#29156,#29157,#29158,#29159,#29160,#29161,#29162),
 .UNSPECIFIED.,.F.,.F.,(4,3,3,3,3,3,3,3,3,3,3,3,3,3,3,3,4),(0.,0.0320358644790656,
0.0566025392350713,0.0661929095230273,0.097524509655756,0.113218578765797,
0.122777613428698,0.148357330195644,0.170686258066526,0.180239221440332,
0.205963417559621,0.220473935588774,0.231002296372473,0.247562418687567,
0.263621625608468,0.283136005917488,0.286347380332233),.UNSPECIFIED.);
#2802=LINE('',#27646,#3376);
#2803=LINE('',#27655,#3377);
#2804=LINE('',#27672,#3378);
#2805=LINE('',#27723,#3379);
#2806=LINE('',#27774,#3380);
#2807=LINE('',#27822,#3381);
#2808=LINE('',#27870,#3382);
#2809=LINE('',#27921,#3383);
#2810=LINE('',#27972,#3384);
#2811=LINE('',#28020,#3385);
#2812=LINE('',#28071,#3386);
#2813=LINE('',#28110,#3387);
#2814=LINE('',#28134,#3388);
#2815=LINE('',#28158,#3389);
#2816=LINE('',#28183,#3390);
#2817=LINE('',#28207,#3391);
#2818=LINE('',#28232,#3392);
#2819=LINE('',#28256,#3393);
#2820=LINE('',#28281,#3394);
#2821=LINE('',#28306,#3395);
#2822=LINE('',#28330,#3396);
#2823=LINE('',#29169,#3397);
#2824=LINE('',#29174,#3398);
#2825=LINE('',#29176,#3399);
#2826=LINE('',#29178,#3400);
#2827=LINE('',#29179,#3401);
#2828=LINE('',#29183,#3402);
#2829=LINE('',#29184,#3403);
#2830=LINE('',#29185,#3404);
#2831=LINE('',#29188,#3405);
#2832=LINE('',#29190,#3406);
#2833=LINE('',#29192,#3407);
#2834=LINE('',#29193,#3408);
#2835=LINE('',#29196,#3409);
#2836=LINE('',#29197,#3410);
#2837=LINE('',#29200,#3411);
#2838=LINE('',#29202,#3412);
#2839=LINE('',#29203,#3413);
#2840=LINE('',#29205,#3414);
#2841=LINE('',#29206,#3415);
#3376=VECTOR('',#11909,0.15);
#3377=VECTOR('',#11912,0.15);
#3378=VECTOR('',#11919,0.15);
#3379=VECTOR('',#11922,0.15);
#3380=VECTOR('',#11925,0.15);
#3381=VECTOR('',#11928,0.15);
#3382=VECTOR('',#11931,0.15);
#3383=VECTOR('',#11934,0.15);
#3384=VECTOR('',#11937,0.15);
#3385=VECTOR('',#11940,0.15);
#3386=VECTOR('',#11943,0.15);
#3387=VECTOR('',#11948,0.1543);
#3388=VECTOR('',#11953,0.1543);
#3389=VECTOR('',#11956,0.1543);
#3390=VECTOR('',#11959,0.1543);
#3391=VECTOR('',#11962,0.1543);
#3392=VECTOR('',#11965,0.1543);
#3393=VECTOR('',#11968,0.1543);
#3394=VECTOR('',#11971,0.1543);
#3395=VECTOR('',#11974,0.1543);
#3396=VECTOR('',#11977,0.1543);
#3397=VECTOR('',#11992,0.2);
#3398=VECTOR('',#11997,1.);
#3399=VECTOR('',#11998,1.);
#3400=VECTOR('',#11999,1.);
#3401=VECTOR('',#12000,1.);
#3402=VECTOR('',#12003,1.);
#3403=VECTOR('',#12004,1.);
#3404=VECTOR('',#12005,1.);
#3405=VECTOR('',#12008,1.);
#3406=VECTOR('',#12009,1.);
#3407=VECTOR('',#12010,1.);
#3408=VECTOR('',#12011,1.);
#3409=VECTOR('',#12014,1.);
#3410=VECTOR('',#12015,1.);
#3411=VECTOR('',#12018,1.);
#3412=VECTOR('',#12019,1.);
#3413=VECTOR('',#12020,1.);
#3414=VECTOR('',#12023,1.);
#3415=VECTOR('',#12024,1.);
#4201=VERTEX_POINT('',#27644);
#4202=VERTEX_POINT('',#27645);
#4203=VERTEX_POINT('',#27647);
#4204=VERTEX_POINT('',#27652);
#4205=VERTEX_POINT('',#27654);
#4206=VERTEX_POINT('',#27657);
#4207=VERTEX_POINT('',#27670);
#4208=VERTEX_POINT('',#27671);
#4209=VERTEX_POINT('',#27721);
#4210=VERTEX_POINT('',#27722);
#4211=VERTEX_POINT('',#27772);
#4212=VERTEX_POINT('',#27773);
#4213=VERTEX_POINT('',#27820);
#4214=VERTEX_POINT('',#27821);
#4215=VERTEX_POINT('',#27868);
#4216=VERTEX_POINT('',#27869);
#4217=VERTEX_POINT('',#27919);
#4218=VERTEX_POINT('',#27920);
#4219=VERTEX_POINT('',#27970);
#4220=VERTEX_POINT('',#27971);
#4221=VERTEX_POINT('',#28018);
#4222=VERTEX_POINT('',#28019);
#4223=VERTEX_POINT('',#28069);
#4224=VERTEX_POINT('',#28070);
#4225=VERTEX_POINT('',#28072);
#4226=VERTEX_POINT('',#28086);
#4227=VERTEX_POINT('',#28108);
#4228=VERTEX_POINT('',#28109);
#4229=VERTEX_POINT('',#28111);
#4230=VERTEX_POINT('',#28120);
#4231=VERTEX_POINT('',#28132);
#4232=VERTEX_POINT('',#28133);
#4233=VERTEX_POINT('',#28156);
#4234=VERTEX_POINT('',#28157);
#4235=VERTEX_POINT('',#28181);
#4236=VERTEX_POINT('',#28182);
#4237=VERTEX_POINT('',#28205);
#4238=VERTEX_POINT('',#28206);
#4239=VERTEX_POINT('',#28230);
#4240=VERTEX_POINT('',#28231);
#4241=VERTEX_POINT('',#28254);
#4242=VERTEX_POINT('',#28255);
#4243=VERTEX_POINT('',#28279);
#4244=VERTEX_POINT('',#28280);
#4245=VERTEX_POINT('',#28304);
#4246=VERTEX_POINT('',#28305);
#4247=VERTEX_POINT('',#28328);
#4248=VERTEX_POINT('',#28329);
#4249=VERTEX_POINT('',#28331);
#4250=VERTEX_POINT('',#28337);
#4251=VERTEX_POINT('',#29166);
#4252=VERTEX_POINT('',#29168);
#4253=VERTEX_POINT('',#29172);
#4254=VERTEX_POINT('',#29173);
#4255=VERTEX_POINT('',#29175);
#4256=VERTEX_POINT('',#29177);
#4257=VERTEX_POINT('',#29181);
#4258=VERTEX_POINT('',#29182);
#4259=VERTEX_POINT('',#29187);
#4260=VERTEX_POINT('',#29189);
#4261=VERTEX_POINT('',#29191);
#4262=VERTEX_POINT('',#29195);
#4263=VERTEX_POINT('',#29199);
#4264=VERTEX_POINT('',#29201);
#5464=EDGE_CURVE('',#4201,#4202,#2802,.T.);
#5465=EDGE_CURVE('',#4202,#4203,#2193,.T.);
#5466=EDGE_CURVE('',#4203,#4204,#1685,.T.);
#5467=EDGE_CURVE('',#4204,#4205,#2803,.T.);
#5468=EDGE_CURVE('',#4205,#4205,#1686,.F.);
#5469=EDGE_CURVE('',#4204,#4206,#1687,.T.);
#5470=EDGE_CURVE('',#4206,#4201,#2194,.T.);
#5471=EDGE_CURVE('',#4207,#4208,#2804,.T.);
#5472=EDGE_CURVE('',#4208,#4202,#2195,.T.);
#5473=EDGE_CURVE('',#4201,#4207,#2196,.T.);
#5474=EDGE_CURVE('',#4209,#4210,#2805,.T.);
#5475=EDGE_CURVE('',#4210,#4208,#2197,.T.);
#5476=EDGE_CURVE('',#4207,#4209,#2198,.T.);
#5477=EDGE_CURVE('',#4211,#4212,#2806,.T.);
#5478=EDGE_CURVE('',#4212,#4210,#2199,.T.);
#5479=EDGE_CURVE('',#4209,#4211,#2200,.T.);
#5480=EDGE_CURVE('',#4213,#4214,#2807,.T.);
#5481=EDGE_CURVE('',#4214,#4212,#2201,.T.);
#5482=EDGE_CURVE('',#4211,#4213,#2202,.T.);
#5483=EDGE_CURVE('',#4215,#4216,#2808,.T.);
#5484=EDGE_CURVE('',#4216,#4214,#2203,.T.);
#5485=EDGE_CURVE('',#4213,#4215,#2204,.T.);
#5486=EDGE_CURVE('',#4217,#4218,#2809,.T.);
#5487=EDGE_CURVE('',#4218,#4216,#2205,.T.);
#5488=EDGE_CURVE('',#4215,#4217,#2206,.T.);
#5489=EDGE_CURVE('',#4219,#4220,#2810,.T.);
#5490=EDGE_CURVE('',#4220,#4218,#2207,.T.);
#5491=EDGE_CURVE('',#4217,#4219,#2208,.T.);
#5492=EDGE_CURVE('',#4221,#4222,#2811,.T.);
#5493=EDGE_CURVE('',#4222,#4220,#2209,.T.);
#5494=EDGE_CURVE('',#4219,#4221,#2210,.T.);
#5495=EDGE_CURVE('',#4223,#4224,#2812,.T.);
#5496=EDGE_CURVE('',#4223,#4225,#2211,.T.);
#5497=EDGE_CURVE('',#4226,#4225,#1688,.T.);
#5498=EDGE_CURVE('',#4226,#4224,#2212,.T.);
#5499=EDGE_CURVE('',#4227,#4228,#2813,.T.);
#5500=EDGE_CURVE('',#4228,#4229,#2213,.T.);
#5501=EDGE_CURVE('',#4230,#4229,#1689,.T.);
#5502=EDGE_CURVE('',#4227,#4230,#2214,.T.);
#5503=EDGE_CURVE('',#4231,#4232,#2814,.T.);
#5504=EDGE_CURVE('',#4232,#4228,#2215,.T.);
#5505=EDGE_CURVE('',#4231,#4227,#2216,.T.);
#5506=EDGE_CURVE('',#4233,#4234,#2815,.T.);
#5507=EDGE_CURVE('',#4234,#4232,#2217,.T.);
#5508=EDGE_CURVE('',#4233,#4231,#2218,.T.);
#5509=EDGE_CURVE('',#4235,#4236,#2816,.T.);
#5510=EDGE_CURVE('',#4236,#4234,#2219,.T.);
#5511=EDGE_CURVE('',#4235,#4233,#2220,.T.);
#5512=EDGE_CURVE('',#4237,#4238,#2817,.T.);
#5513=EDGE_CURVE('',#4238,#4236,#2221,.T.);
#5514=EDGE_CURVE('',#4237,#4235,#2222,.T.);
#5515=EDGE_CURVE('',#4239,#4240,#2818,.T.);
#5516=EDGE_CURVE('',#4240,#4238,#2223,.T.);
#5517=EDGE_CURVE('',#4239,#4237,#2224,.T.);
#5518=EDGE_CURVE('',#4241,#4242,#2819,.T.);
#5519=EDGE_CURVE('',#4242,#4240,#2225,.T.);
#5520=EDGE_CURVE('',#4241,#4239,#2226,.T.);
#5521=EDGE_CURVE('',#4243,#4244,#2820,.T.);
#5522=EDGE_CURVE('',#4244,#4242,#2227,.T.);
#5523=EDGE_CURVE('',#4243,#4241,#2228,.T.);
#5524=EDGE_CURVE('',#4245,#4246,#2821,.T.);
#5525=EDGE_CURVE('',#4246,#4244,#2229,.T.);
#5526=EDGE_CURVE('',#4245,#4243,#2230,.T.);
#5527=EDGE_CURVE('',#4247,#4248,#2822,.T.);
#5528=EDGE_CURVE('',#4249,#4247,#2231,.T.);
#5529=EDGE_CURVE('',#4250,#4249,#1690,.T.);
#5530=EDGE_CURVE('',#4250,#4248,#2232,.T.);
#5531=EDGE_CURVE('',#4203,#4230,#2233,.T.);
#5532=EDGE_CURVE('',#4229,#4206,#2234,.T.);
#5533=EDGE_CURVE('',#4248,#4246,#2235,.T.);
#5534=EDGE_CURVE('',#4247,#4245,#2236,.T.);
#5535=EDGE_CURVE('',#4225,#4250,#2237,.T.);
#5536=EDGE_CURVE('',#4221,#4223,#2238,.T.);
#5537=EDGE_CURVE('',#4224,#4222,#2239,.T.);
#5538=EDGE_CURVE('',#4249,#4226,#2240,.T.);
#5539=EDGE_CURVE('',#4251,#4251,#1691,.T.);
#5540=EDGE_CURVE('',#4251,#4252,#2823,.T.);
#5541=EDGE_CURVE('',#4252,#4252,#1692,.T.);
#5542=EDGE_CURVE('',#4253,#4254,#2824,.T.);
#5543=EDGE_CURVE('',#4254,#4255,#2825,.T.);
#5544=EDGE_CURVE('',#4256,#4255,#2826,.T.);
#5545=EDGE_CURVE('',#4253,#4256,#2827,.T.);
#5546=EDGE_CURVE('',#4257,#4258,#2828,.T.);
#5547=EDGE_CURVE('',#4254,#4257,#2829,.T.);
#5548=EDGE_CURVE('',#4258,#4253,#2830,.T.);
#5549=EDGE_CURVE('',#4255,#4259,#2831,.T.);
#5550=EDGE_CURVE('',#4260,#4257,#2832,.T.);
#5551=EDGE_CURVE('',#4260,#4261,#2833,.T.);
#5552=EDGE_CURVE('',#4261,#4259,#2834,.T.);
#5553=EDGE_CURVE('',#4262,#4258,#2835,.T.);
#5554=EDGE_CURVE('',#4262,#4260,#2836,.T.);
#5555=EDGE_CURVE('',#4263,#4256,#2837,.T.);
#5556=EDGE_CURVE('',#4264,#4263,#2838,.T.);
#5557=EDGE_CURVE('',#4264,#4262,#2839,.T.);
#5558=EDGE_CURVE('',#4261,#4264,#2840,.T.);
#5559=EDGE_CURVE('',#4259,#4263,#2841,.T.);
#7816=ORIENTED_EDGE('',*,*,#5464,.T.);
#7817=ORIENTED_EDGE('',*,*,#5465,.T.);
#7818=ORIENTED_EDGE('',*,*,#5466,.T.);
#7819=ORIENTED_EDGE('',*,*,#5467,.T.);
#7820=ORIENTED_EDGE('',*,*,#5468,.T.);
#7821=ORIENTED_EDGE('',*,*,#5467,.F.);
#7822=ORIENTED_EDGE('',*,*,#5469,.T.);
#7823=ORIENTED_EDGE('',*,*,#5470,.T.);
#7824=ORIENTED_EDGE('',*,*,#5471,.T.);
#7825=ORIENTED_EDGE('',*,*,#5472,.T.);
#7826=ORIENTED_EDGE('',*,*,#5464,.F.);
#7827=ORIENTED_EDGE('',*,*,#5473,.T.);
#7828=ORIENTED_EDGE('',*,*,#5474,.T.);
#7829=ORIENTED_EDGE('',*,*,#5475,.T.);
#7830=ORIENTED_EDGE('',*,*,#5471,.F.);
#7831=ORIENTED_EDGE('',*,*,#5476,.T.);
#7832=ORIENTED_EDGE('',*,*,#5477,.T.);
#7833=ORIENTED_EDGE('',*,*,#5478,.T.);
#7834=ORIENTED_EDGE('',*,*,#5474,.F.);
#7835=ORIENTED_EDGE('',*,*,#5479,.T.);
#7836=ORIENTED_EDGE('',*,*,#5480,.T.);
#7837=ORIENTED_EDGE('',*,*,#5481,.T.);
#7838=ORIENTED_EDGE('',*,*,#5477,.F.);
#7839=ORIENTED_EDGE('',*,*,#5482,.T.);
#7840=ORIENTED_EDGE('',*,*,#5483,.T.);
#7841=ORIENTED_EDGE('',*,*,#5484,.T.);
#7842=ORIENTED_EDGE('',*,*,#5480,.F.);
#7843=ORIENTED_EDGE('',*,*,#5485,.T.);
#7844=ORIENTED_EDGE('',*,*,#5486,.T.);
#7845=ORIENTED_EDGE('',*,*,#5487,.T.);
#7846=ORIENTED_EDGE('',*,*,#5483,.F.);
#7847=ORIENTED_EDGE('',*,*,#5488,.T.);
#7848=ORIENTED_EDGE('',*,*,#5489,.T.);
#7849=ORIENTED_EDGE('',*,*,#5490,.T.);
#7850=ORIENTED_EDGE('',*,*,#5486,.F.);
#7851=ORIENTED_EDGE('',*,*,#5491,.T.);
#7852=ORIENTED_EDGE('',*,*,#5492,.T.);
#7853=ORIENTED_EDGE('',*,*,#5493,.T.);
#7854=ORIENTED_EDGE('',*,*,#5489,.F.);
#7855=ORIENTED_EDGE('',*,*,#5494,.T.);
#7856=ORIENTED_EDGE('',*,*,#5495,.F.);
#7857=ORIENTED_EDGE('',*,*,#5496,.T.);
#7858=ORIENTED_EDGE('',*,*,#5497,.F.);
#7859=ORIENTED_EDGE('',*,*,#5498,.T.);
#7860=ORIENTED_EDGE('',*,*,#5499,.T.);
#7861=ORIENTED_EDGE('',*,*,#5500,.T.);
#7862=ORIENTED_EDGE('',*,*,#5501,.F.);
#7863=ORIENTED_EDGE('',*,*,#5502,.F.);
#7864=ORIENTED_EDGE('',*,*,#5503,.T.);
#7865=ORIENTED_EDGE('',*,*,#5504,.T.);
#7866=ORIENTED_EDGE('',*,*,#5499,.F.);
#7867=ORIENTED_EDGE('',*,*,#5505,.F.);
#7868=ORIENTED_EDGE('',*,*,#5506,.T.);
#7869=ORIENTED_EDGE('',*,*,#5507,.T.);
#7870=ORIENTED_EDGE('',*,*,#5503,.F.);
#7871=ORIENTED_EDGE('',*,*,#5508,.F.);
#7872=ORIENTED_EDGE('',*,*,#5509,.T.);
#7873=ORIENTED_EDGE('',*,*,#5510,.T.);
#7874=ORIENTED_EDGE('',*,*,#5506,.F.);
#7875=ORIENTED_EDGE('',*,*,#5511,.F.);
#7876=ORIENTED_EDGE('',*,*,#5512,.T.);
#7877=ORIENTED_EDGE('',*,*,#5513,.T.);
#7878=ORIENTED_EDGE('',*,*,#5509,.F.);
#7879=ORIENTED_EDGE('',*,*,#5514,.F.);
#7880=ORIENTED_EDGE('',*,*,#5515,.T.);
#7881=ORIENTED_EDGE('',*,*,#5516,.T.);
#7882=ORIENTED_EDGE('',*,*,#5512,.F.);
#7883=ORIENTED_EDGE('',*,*,#5517,.F.);
#7884=ORIENTED_EDGE('',*,*,#5518,.T.);
#7885=ORIENTED_EDGE('',*,*,#5519,.T.);
#7886=ORIENTED_EDGE('',*,*,#5515,.F.);
#7887=ORIENTED_EDGE('',*,*,#5520,.F.);
#7888=ORIENTED_EDGE('',*,*,#5521,.T.);
#7889=ORIENTED_EDGE('',*,*,#5522,.T.);
#7890=ORIENTED_EDGE('',*,*,#5518,.F.);
#7891=ORIENTED_EDGE('',*,*,#5523,.F.);
#7892=ORIENTED_EDGE('',*,*,#5524,.T.);
#7893=ORIENTED_EDGE('',*,*,#5525,.T.);
#7894=ORIENTED_EDGE('',*,*,#5521,.F.);
#7895=ORIENTED_EDGE('',*,*,#5526,.F.);
#7896=ORIENTED_EDGE('',*,*,#5527,.F.);
#7897=ORIENTED_EDGE('',*,*,#5528,.F.);
#7898=ORIENTED_EDGE('',*,*,#5529,.F.);
#7899=ORIENTED_EDGE('',*,*,#5530,.T.);
#7900=ORIENTED_EDGE('',*,*,#5466,.F.);
#7901=ORIENTED_EDGE('',*,*,#5531,.T.);
#7902=ORIENTED_EDGE('',*,*,#5501,.T.);
#7903=ORIENTED_EDGE('',*,*,#5532,.T.);
#7904=ORIENTED_EDGE('',*,*,#5469,.F.);
#7905=ORIENTED_EDGE('',*,*,#5527,.T.);
#7906=ORIENTED_EDGE('',*,*,#5533,.T.);
#7907=ORIENTED_EDGE('',*,*,#5524,.F.);
#7908=ORIENTED_EDGE('',*,*,#5534,.F.);
#7909=ORIENTED_EDGE('',*,*,#5532,.F.);
#7910=ORIENTED_EDGE('',*,*,#5500,.F.);
#7911=ORIENTED_EDGE('',*,*,#5504,.F.);
#7912=ORIENTED_EDGE('',*,*,#5507,.F.);
#7913=ORIENTED_EDGE('',*,*,#5510,.F.);
#7914=ORIENTED_EDGE('',*,*,#5513,.F.);
#7915=ORIENTED_EDGE('',*,*,#5516,.F.);
#7916=ORIENTED_EDGE('',*,*,#5519,.F.);
#7917=ORIENTED_EDGE('',*,*,#5522,.F.);
#7918=ORIENTED_EDGE('',*,*,#5525,.F.);
#7919=ORIENTED_EDGE('',*,*,#5533,.F.);
#7920=ORIENTED_EDGE('',*,*,#5530,.F.);
#7921=ORIENTED_EDGE('',*,*,#5535,.F.);
#7922=ORIENTED_EDGE('',*,*,#5496,.F.);
#7923=ORIENTED_EDGE('',*,*,#5536,.F.);
#7924=ORIENTED_EDGE('',*,*,#5494,.F.);
#7925=ORIENTED_EDGE('',*,*,#5491,.F.);
#7926=ORIENTED_EDGE('',*,*,#5488,.F.);
#7927=ORIENTED_EDGE('',*,*,#5485,.F.);
#7928=ORIENTED_EDGE('',*,*,#5482,.F.);
#7929=ORIENTED_EDGE('',*,*,#5479,.F.);
#7930=ORIENTED_EDGE('',*,*,#5476,.F.);
#7931=ORIENTED_EDGE('',*,*,#5473,.F.);
#7932=ORIENTED_EDGE('',*,*,#5470,.F.);
#7933=ORIENTED_EDGE('',*,*,#5531,.F.);
#7934=ORIENTED_EDGE('',*,*,#5465,.F.);
#7935=ORIENTED_EDGE('',*,*,#5472,.F.);
#7936=ORIENTED_EDGE('',*,*,#5475,.F.);
#7937=ORIENTED_EDGE('',*,*,#5478,.F.);
#7938=ORIENTED_EDGE('',*,*,#5481,.F.);
#7939=ORIENTED_EDGE('',*,*,#5484,.F.);
#7940=ORIENTED_EDGE('',*,*,#5487,.F.);
#7941=ORIENTED_EDGE('',*,*,#5490,.F.);
#7942=ORIENTED_EDGE('',*,*,#5493,.F.);
#7943=ORIENTED_EDGE('',*,*,#5537,.F.);
#7944=ORIENTED_EDGE('',*,*,#5498,.F.);
#7945=ORIENTED_EDGE('',*,*,#5538,.F.);
#7946=ORIENTED_EDGE('',*,*,#5528,.T.);
#7947=ORIENTED_EDGE('',*,*,#5534,.T.);
#7948=ORIENTED_EDGE('',*,*,#5526,.T.);
#7949=ORIENTED_EDGE('',*,*,#5523,.T.);
#7950=ORIENTED_EDGE('',*,*,#5520,.T.);
#7951=ORIENTED_EDGE('',*,*,#5517,.T.);
#7952=ORIENTED_EDGE('',*,*,#5514,.T.);
#7953=ORIENTED_EDGE('',*,*,#5511,.T.);
#7954=ORIENTED_EDGE('',*,*,#5508,.T.);
#7955=ORIENTED_EDGE('',*,*,#5505,.T.);
#7956=ORIENTED_EDGE('',*,*,#5502,.T.);
#7957=ORIENTED_EDGE('',*,*,#5495,.T.);
#7958=ORIENTED_EDGE('',*,*,#5537,.T.);
#7959=ORIENTED_EDGE('',*,*,#5492,.F.);
#7960=ORIENTED_EDGE('',*,*,#5536,.T.);
#7961=ORIENTED_EDGE('',*,*,#5468,.F.);
#7962=ORIENTED_EDGE('',*,*,#5539,.F.);
#7963=ORIENTED_EDGE('',*,*,#5540,.T.);
#7964=ORIENTED_EDGE('',*,*,#5541,.F.);
#7965=ORIENTED_EDGE('',*,*,#5540,.F.);
#7966=ORIENTED_EDGE('',*,*,#5542,.T.);
#7967=ORIENTED_EDGE('',*,*,#5543,.T.);
#7968=ORIENTED_EDGE('',*,*,#5544,.F.);
#7969=ORIENTED_EDGE('',*,*,#5545,.F.);
#7970=ORIENTED_EDGE('',*,*,#5546,.F.);
#7971=ORIENTED_EDGE('',*,*,#5547,.F.);
#7972=ORIENTED_EDGE('',*,*,#5542,.F.);
#7973=ORIENTED_EDGE('',*,*,#5548,.F.);
#7974=ORIENTED_EDGE('',*,*,#5541,.T.);
#7975=ORIENTED_EDGE('',*,*,#5549,.F.);
#7976=ORIENTED_EDGE('',*,*,#5543,.F.);
#7977=ORIENTED_EDGE('',*,*,#5547,.T.);
#7978=ORIENTED_EDGE('',*,*,#5550,.F.);
#7979=ORIENTED_EDGE('',*,*,#5551,.T.);
#7980=ORIENTED_EDGE('',*,*,#5552,.T.);
#7981=ORIENTED_EDGE('',*,*,#5546,.T.);
#7982=ORIENTED_EDGE('',*,*,#5553,.F.);
#7983=ORIENTED_EDGE('',*,*,#5554,.T.);
#7984=ORIENTED_EDGE('',*,*,#5550,.T.);
#7985=ORIENTED_EDGE('',*,*,#5555,.F.);
#7986=ORIENTED_EDGE('',*,*,#5556,.F.);
#7987=ORIENTED_EDGE('',*,*,#5557,.T.);
#7988=ORIENTED_EDGE('',*,*,#5553,.T.);
#7989=ORIENTED_EDGE('',*,*,#5548,.T.);
#7990=ORIENTED_EDGE('',*,*,#5545,.T.);
#7991=ORIENTED_EDGE('',*,*,#5558,.T.);
#7992=ORIENTED_EDGE('',*,*,#5556,.T.);
#7993=ORIENTED_EDGE('',*,*,#5559,.F.);
#7994=ORIENTED_EDGE('',*,*,#5552,.F.);
#7995=ORIENTED_EDGE('',*,*,#5549,.T.);
#7996=ORIENTED_EDGE('',*,*,#5559,.T.);
#7997=ORIENTED_EDGE('',*,*,#5555,.T.);
#7998=ORIENTED_EDGE('',*,*,#5544,.T.);
#7999=ORIENTED_EDGE('',*,*,#5538,.T.);
#8000=ORIENTED_EDGE('',*,*,#5497,.T.);
#8001=ORIENTED_EDGE('',*,*,#5535,.T.);
#8002=ORIENTED_EDGE('',*,*,#5529,.T.);
#8003=ORIENTED_EDGE('',*,*,#5539,.T.);
#8004=ORIENTED_EDGE('',*,*,#5558,.F.);
#8005=ORIENTED_EDGE('',*,*,#5551,.F.);
#8006=ORIENTED_EDGE('',*,*,#5554,.F.);
#8007=ORIENTED_EDGE('',*,*,#5557,.F.);
#9098=CYLINDRICAL_SURFACE('',#10402,0.12645);
#9099=CYLINDRICAL_SURFACE('',#10406,0.12645);
#9100=CYLINDRICAL_SURFACE('',#10407,0.12645);
#9101=CYLINDRICAL_SURFACE('',#10408,0.12645);
#9102=CYLINDRICAL_SURFACE('',#10409,0.12645);
#9103=CYLINDRICAL_SURFACE('',#10410,0.12645);
#9104=CYLINDRICAL_SURFACE('',#10411,0.12645);
#9105=CYLINDRICAL_SURFACE('',#10412,0.12645);
#9106=CYLINDRICAL_SURFACE('',#10413,0.12645);
#9107=CYLINDRICAL_SURFACE('',#10414,0.12645);
#9108=CYLINDRICAL_SURFACE('',#10416,0.1543);
#9109=CYLINDRICAL_SURFACE('',#10418,0.1543);
#9110=CYLINDRICAL_SURFACE('',#10419,0.1543);
#9111=CYLINDRICAL_SURFACE('',#10420,0.1543);
#9112=CYLINDRICAL_SURFACE('',#10421,0.1543);
#9113=CYLINDRICAL_SURFACE('',#10422,0.1543);
#9114=CYLINDRICAL_SURFACE('',#10423,0.1543);
#9115=CYLINDRICAL_SURFACE('',#10424,0.1543);
#9116=CYLINDRICAL_SURFACE('',#10425,0.1543);
#9117=CYLINDRICAL_SURFACE('',#10426,0.1543);
#9118=CYLINDRICAL_SURFACE('',#10429,0.1543);
#9119=CYLINDRICAL_SURFACE('',#10430,0.12645);
#9120=CYLINDRICAL_SURFACE('',#10432,0.2);
#9563=ADVANCED_FACE('',(#773),#9098,.F.);
#9564=ADVANCED_FACE('',(#774),#9099,.F.);
#9565=ADVANCED_FACE('',(#775),#9100,.F.);
#9566=ADVANCED_FACE('',(#776),#9101,.F.);
#9567=ADVANCED_FACE('',(#777),#9102,.F.);
#9568=ADVANCED_FACE('',(#778),#9103,.F.);
#9569=ADVANCED_FACE('',(#779),#9104,.F.);
#9570=ADVANCED_FACE('',(#780),#9105,.F.);
#9571=ADVANCED_FACE('',(#781),#9106,.F.);
#9572=ADVANCED_FACE('',(#782),#9107,.F.);
#9573=ADVANCED_FACE('',(#783),#9108,.F.);
#9574=ADVANCED_FACE('',(#784),#9109,.F.);
#9575=ADVANCED_FACE('',(#785),#9110,.F.);
#9576=ADVANCED_FACE('',(#786),#9111,.F.);
#9577=ADVANCED_FACE('',(#787),#9112,.F.);
#9578=ADVANCED_FACE('',(#788),#9113,.F.);
#9579=ADVANCED_FACE('',(#789),#9114,.F.);
#9580=ADVANCED_FACE('',(#790),#9115,.F.);
#9581=ADVANCED_FACE('',(#791),#9116,.F.);
#9582=ADVANCED_FACE('',(#792),#9117,.F.);
#9583=ADVANCED_FACE('',(#793),#378,.T.);
#9584=ADVANCED_FACE('',(#794),#9118,.F.);
#9585=ADVANCED_FACE('',(#795),#226,.F.);
#9586=ADVANCED_FACE('',(#796),#227,.F.);
#9587=ADVANCED_FACE('',(#797),#9119,.F.);
#9588=ADVANCED_FACE('',(#798),#379,.F.);
#9589=ADVANCED_FACE('',(#799),#9120,.F.);
#9590=ADVANCED_FACE('',(#800),#380,.T.);
#9591=ADVANCED_FACE('',(#801,#284),#381,.F.);
#9592=ADVANCED_FACE('',(#802),#382,.T.);
#9593=ADVANCED_FACE('',(#803),#383,.T.);
#9594=ADVANCED_FACE('',(#804),#384,.T.);
#9595=ADVANCED_FACE('',(#805),#385,.T.);
#9596=ADVANCED_FACE('',(#806,#285,#286),#386,.T.);
#9597=ADVANCED_FACE('',(#807),#387,.F.);
#9774=CLOSED_SHELL('',(#9563,#9564,#9565,#9566,#9567,#9568,#9569,#9570,
#9571,#9572,#9573,#9574,#9575,#9576,#9577,#9578,#9579,#9580,#9581,#9582,
#9583,#9584,#9585,#9586,#9587,#9588,#9589,#9590,#9591,#9592,#9593,#9594,
#9595,#9596,#9597));
#10401=AXIS2_PLACEMENT_3D('',#27642,#11905,#11906);
#10402=AXIS2_PLACEMENT_3D('',#27643,#11907,#11908);
#10403=AXIS2_PLACEMENT_3D('',#27653,#11910,#11911);
#10404=AXIS2_PLACEMENT_3D('',#27656,#11913,#11914);
#10405=AXIS2_PLACEMENT_3D('',#27658,#11915,#11916);
#10406=AXIS2_PLACEMENT_3D('',#27669,#11917,#11918);
#10407=AXIS2_PLACEMENT_3D('',#27720,#11920,#11921);
#10408=AXIS2_PLACEMENT_3D('',#27771,#11923,#11924);
#10409=AXIS2_PLACEMENT_3D('',#27819,#11926,#11927);
#10410=AXIS2_PLACEMENT_3D('',#27867,#11929,#11930);
#10411=AXIS2_PLACEMENT_3D('',#27918,#11932,#11933);
#10412=AXIS2_PLACEMENT_3D('',#27969,#11935,#11936);
#10413=AXIS2_PLACEMENT_3D('',#28017,#11938,#11939);
#10414=AXIS2_PLACEMENT_3D('',#28068,#11941,#11942);
#10415=AXIS2_PLACEMENT_3D('',#28087,#11944,#11945);
#10416=AXIS2_PLACEMENT_3D('',#28107,#11946,#11947);
#10417=AXIS2_PLACEMENT_3D('',#28121,#11949,#11950);
#10418=AXIS2_PLACEMENT_3D('',#28131,#11951,#11952);
#10419=AXIS2_PLACEMENT_3D('',#28155,#11954,#11955);
#10420=AXIS2_PLACEMENT_3D('',#28180,#11957,#11958);
#10421=AXIS2_PLACEMENT_3D('',#28204,#11960,#11961);
#10422=AXIS2_PLACEMENT_3D('',#28229,#11963,#11964);
#10423=AXIS2_PLACEMENT_3D('',#28253,#11966,#11967);
#10424=AXIS2_PLACEMENT_3D('',#28278,#11969,#11970);
#10425=AXIS2_PLACEMENT_3D('',#28303,#11972,#11973);
#10426=AXIS2_PLACEMENT_3D('',#28327,#11975,#11976);
#10427=AXIS2_PLACEMENT_3D('',#28338,#11978,#11979);
#10428=AXIS2_PLACEMENT_3D('',#28344,#11980,#11981);
#10429=AXIS2_PLACEMENT_3D('',#28452,#11982,#11983);
#10430=AXIS2_PLACEMENT_3D('',#29163,#11984,#11985);
#10431=AXIS2_PLACEMENT_3D('',#29164,#11986,#11987);
#10432=AXIS2_PLACEMENT_3D('',#29165,#11988,#11989);
#10433=AXIS2_PLACEMENT_3D('',#29167,#11990,#11991);
#10434=AXIS2_PLACEMENT_3D('',#29170,#11993,#11994);
#10435=AXIS2_PLACEMENT_3D('',#29171,#11995,#11996);
#10436=AXIS2_PLACEMENT_3D('',#29180,#12001,#12002);
#10437=AXIS2_PLACEMENT_3D('',#29186,#12006,#12007);
#10438=AXIS2_PLACEMENT_3D('',#29194,#12012,#12013);
#10439=AXIS2_PLACEMENT_3D('',#29198,#12016,#12017);
#10440=AXIS2_PLACEMENT_3D('',#29204,#12021,#12022);
#10441=AXIS2_PLACEMENT_3D('',#29207,#12025,#12026);
#10442=AXIS2_PLACEMENT_3D('',#29208,#12027,#12028);
#11905=DIRECTION('axis',(0.,0.,1.));
#11906=DIRECTION('refdir',(1.,0.,0.));
#11907=DIRECTION('center_axis',(0.,0.,-1.));
#11908=DIRECTION('ref_axis',(1.,0.,0.));
#11909=DIRECTION('',(0.,0.,-1.));
#11910=DIRECTION('center_axis',(0.,0.,1.));
#11911=DIRECTION('ref_axis',(1.,0.,0.));
#11912=DIRECTION('',(0.,0.,-1.));
#11913=DIRECTION('center_axis',(0.,0.,1.));
#11914=DIRECTION('ref_axis',(1.,0.,0.));
#11915=DIRECTION('center_axis',(0.,0.,1.));
#11916=DIRECTION('ref_axis',(1.,0.,0.));
#11917=DIRECTION('center_axis',(0.,0.,-1.));
#11918=DIRECTION('ref_axis',(1.,0.,0.));
#11919=DIRECTION('',(0.,0.,-1.));
#11920=DIRECTION('center_axis',(0.,0.,-1.));
#11921=DIRECTION('ref_axis',(1.,0.,0.));
#11922=DIRECTION('',(0.,0.,-1.));
#11923=DIRECTION('center_axis',(0.,0.,-1.));
#11924=DIRECTION('ref_axis',(1.,0.,0.));
#11925=DIRECTION('',(0.,0.,-1.));
#11926=DIRECTION('center_axis',(0.,0.,-1.));
#11927=DIRECTION('ref_axis',(1.,0.,0.));
#11928=DIRECTION('',(0.,0.,-1.));
#11929=DIRECTION('center_axis',(0.,0.,-1.));
#11930=DIRECTION('ref_axis',(1.,0.,0.));
#11931=DIRECTION('',(0.,0.,-1.));
#11932=DIRECTION('center_axis',(0.,0.,-1.));
#11933=DIRECTION('ref_axis',(1.,0.,0.));
#11934=DIRECTION('',(0.,0.,-1.));
#11935=DIRECTION('center_axis',(0.,0.,-1.));
#11936=DIRECTION('ref_axis',(1.,0.,0.));
#11937=DIRECTION('',(0.,0.,-1.));
#11938=DIRECTION('center_axis',(0.,0.,-1.));
#11939=DIRECTION('ref_axis',(1.,0.,0.));
#11940=DIRECTION('',(0.,0.,-1.));
#11941=DIRECTION('center_axis',(0.,0.,-1.));
#11942=DIRECTION('ref_axis',(0.937367309351136,-0.348342543137946,0.));
#11943=DIRECTION('',(0.,0.,-1.));
#11944=DIRECTION('center_axis',(0.,0.,-1.));
#11945=DIRECTION('ref_axis',(1.,0.,0.));
#11946=DIRECTION('center_axis',(0.,0.,-1.));
#11947=DIRECTION('ref_axis',(1.,-4.8329028703551E-14,0.));
#11948=DIRECTION('',(1.22464679914735E-16,-5.93359662859705E-30,-1.));
#11949=DIRECTION('center_axis',(0.,0.,1.));
#11950=DIRECTION('ref_axis',(1.,-4.8329028703551E-14,0.));
#11951=DIRECTION('center_axis',(0.,0.,-1.));
#11952=DIRECTION('ref_axis',(1.,-4.8329028703551E-14,0.));
#11953=DIRECTION('',(1.22464679914735E-16,-5.93359662859705E-30,-1.));
#11954=DIRECTION('center_axis',(0.,0.,-1.));
#11955=DIRECTION('ref_axis',(1.,-4.8329028703551E-14,0.));
#11956=DIRECTION('',(1.22464679914735E-16,-5.93359662859705E-30,-1.));
#11957=DIRECTION('center_axis',(0.,0.,-1.));
#11958=DIRECTION('ref_axis',(1.,-4.8329028703551E-14,0.));
#11959=DIRECTION('',(1.22464679914735E-16,-5.93359662859705E-30,-1.));
#11960=DIRECTION('center_axis',(0.,0.,-1.));
#11961=DIRECTION('ref_axis',(1.,-4.8329028703551E-14,0.));
#11962=DIRECTION('',(1.22464679914735E-16,-5.93359662859705E-30,-1.));
#11963=DIRECTION('center_axis',(0.,0.,-1.));
#11964=DIRECTION('ref_axis',(1.,-4.8329028703551E-14,0.));
#11965=DIRECTION('',(1.22464679914735E-16,-5.93359662859705E-30,-1.));
#11966=DIRECTION('center_axis',(0.,0.,-1.));
#11967=DIRECTION('ref_axis',(1.,-4.8329028703551E-14,0.));
#11968=DIRECTION('',(1.22464679914735E-16,-5.93359662859705E-30,-1.));
#11969=DIRECTION('center_axis',(0.,0.,-1.));
#11970=DIRECTION('ref_axis',(1.,-4.8329028703551E-14,0.));
#11971=DIRECTION('',(1.22464679914735E-16,-5.93359662859705E-30,-1.));
#11972=DIRECTION('center_axis',(0.,0.,-1.));
#11973=DIRECTION('ref_axis',(1.,-4.8329028703551E-14,0.));
#11974=DIRECTION('',(1.22464679914735E-16,-5.93359662859705E-30,-1.));
#11975=DIRECTION('center_axis',(0.,0.,-1.));
#11976=DIRECTION('ref_axis',(-0.609222020738255,-0.792999703308644,0.));
#11977=DIRECTION('',(1.22464679914735E-16,-5.93359662859705E-30,-1.));
#11978=DIRECTION('center_axis',(0.,0.,-1.));
#11979=DIRECTION('ref_axis',(1.,-4.8329028703551E-14,0.));
#11980=DIRECTION('center_axis',(0.,0.,1.));
#11981=DIRECTION('ref_axis',(1.,0.,0.));
#11982=DIRECTION('center_axis',(0.,0.,-1.));
#11983=DIRECTION('ref_axis',(1.,-4.8329028703551E-14,0.));
#11984=DIRECTION('center_axis',(0.,0.,-1.));
#11985=DIRECTION('ref_axis',(1.,0.,0.));
#11986=DIRECTION('center_axis',(0.,0.,-1.));
#11987=DIRECTION('ref_axis',(1.,0.,0.));
#11988=DIRECTION('center_axis',(0.,0.,-1.));
#11989=DIRECTION('ref_axis',(1.,0.,0.));
#11990=DIRECTION('center_axis',(0.,0.,-1.));
#11991=DIRECTION('ref_axis',(1.,0.,0.));
#11992=DIRECTION('',(0.,0.,-1.));
#11993=DIRECTION('center_axis',(0.,0.,1.));
#11994=DIRECTION('ref_axis',(1.,0.,0.));
#11995=DIRECTION('center_axis',(1.,0.,0.));
#11996=DIRECTION('ref_axis',(0.,1.,0.));
#11997=DIRECTION('',(0.,1.,0.));
#11998=DIRECTION('',(0.,0.,1.));
#11999=DIRECTION('',(0.,1.,0.));
#12000=DIRECTION('',(0.,0.,1.));
#12001=DIRECTION('center_axis',(0.,0.,1.));
#12002=DIRECTION('ref_axis',(1.,0.,0.));
#12003=DIRECTION('',(0.,-1.,0.));
#12004=DIRECTION('',(-1.,0.,0.));
#12005=DIRECTION('',(1.,0.,0.));
#12006=DIRECTION('center_axis',(0.,1.,0.));
#12007=DIRECTION('ref_axis',(-1.,0.,0.));
#12008=DIRECTION('',(-1.,0.,0.));
#12009=DIRECTION('',(0.,0.,1.));
#12010=DIRECTION('',(-1.,0.,0.));
#12011=DIRECTION('',(0.,0.,1.));
#12012=DIRECTION('center_axis',(1.,0.,0.));
#12013=DIRECTION('ref_axis',(0.,1.,0.));
#12014=DIRECTION('',(0.,0.,1.));
#12015=DIRECTION('',(0.,1.,0.));
#12016=DIRECTION('center_axis',(0.,-1.,0.));
#12017=DIRECTION('ref_axis',(1.,0.,0.));
#12018=DIRECTION('',(1.,0.,0.));
#12019=DIRECTION('',(0.,0.,1.));
#12020=DIRECTION('',(1.,0.,0.));
#12021=DIRECTION('center_axis',(-1.,0.,0.));
#12022=DIRECTION('ref_axis',(0.,-1.,0.));
#12023=DIRECTION('',(0.,-1.,0.));
#12024=DIRECTION('',(0.,-1.,0.));
#12025=DIRECTION('center_axis',(0.,0.,1.));
#12026=DIRECTION('ref_axis',(1.,0.,0.));
#12027=DIRECTION('center_axis',(0.,0.,1.));
#12028=DIRECTION('ref_axis',(1.,0.,0.));
#27642=CARTESIAN_POINT('',(0.,0.,0.));
#27643=CARTESIAN_POINT('Origin',(0.,0.,3.7));
#27644=CARTESIAN_POINT('',(-0.126245375007135,3.12536796039931E-5,3.51934196736194));
#27645=CARTESIAN_POINT('',(-0.126365398388193,-0.00016976464794081,3.50565803263806));
#27646=CARTESIAN_POINT('',(-0.12645,1.54856587752183E-17,3.7));
#27647=CARTESIAN_POINT('',(-0.0958116152722475,0.0825211298936389,3.5));
#27648=CARTESIAN_POINT('Ctrl Pts',(-0.126365398388193,-0.00016976464794081,
3.50565803263806));
#27649=CARTESIAN_POINT('Ctrl Pts',(-0.126096583499468,0.0297434857833807,
3.5037720217587));
#27650=CARTESIAN_POINT('Ctrl Pts',(-0.115369380269343,0.0598134784363466,
3.50188601087935));
#27651=CARTESIAN_POINT('Ctrl Pts',(-0.0958116152722475,0.0825211298936389,
3.5));
#27652=CARTESIAN_POINT('',(-0.12645,1.54856587752183E-17,3.5));
#27653=CARTESIAN_POINT('Origin',(0.,0.,3.5));
#27654=CARTESIAN_POINT('',(-0.12645,-1.54856587752183E-17,3.4));
#27655=CARTESIAN_POINT('',(-0.12645,1.54856587752183E-17,3.7));
#27656=CARTESIAN_POINT('Origin',(0.,0.,3.4));
#27657=CARTESIAN_POINT('',(0.095993992990581,0.0826600147079878,3.5));
#27658=CARTESIAN_POINT('Origin',(0.,0.,3.5));
#27659=CARTESIAN_POINT('Ctrl Pts',(0.0959941578858439,0.0826601402795114,
3.5));
#27660=CARTESIAN_POINT('Ctrl Pts',(0.0693049284490514,0.113544181600847,
3.5025799450779));
#27661=CARTESIAN_POINT('Ctrl Pts',(0.0262885066473286,0.130447374694629,
3.5051598901558));
#27662=CARTESIAN_POINT('Ctrl Pts',(-0.0142676563835003,0.125842979166089,
3.5077398352337));
#27663=CARTESIAN_POINT('Ctrl Pts',(-0.0558709915822301,0.121119696778261,
3.51038639525932));
#27664=CARTESIAN_POINT('Ctrl Pts',(-0.0948853785622285,0.0937638222778825,
3.51303295528495));
#27665=CARTESIAN_POINT('Ctrl Pts',(-0.113475688700545,0.0562620506672719,
3.51567951531057));
#27666=CARTESIAN_POINT('Ctrl Pts',(-0.122051112249405,0.0389630614088429,
3.51690033266103));
#27667=CARTESIAN_POINT('Ctrl Pts',(-0.126280629837482,0.0195051929476654,
3.51812115001148));
#27668=CARTESIAN_POINT('Ctrl Pts',(-0.126245375007135,3.12536796039931E-5,
3.51934196736194));
#27669=CARTESIAN_POINT('Origin',(0.,0.,3.7));
#27670=CARTESIAN_POINT('',(-0.126440375727766,-0.00011573372396179,3.56934196736194));
#27671=CARTESIAN_POINT('',(-0.126657922659285,8.80032312977707E-6,3.55565803263806));
#27672=CARTESIAN_POINT('',(-0.12645,1.54856587752183E-17,3.7));
#27673=CARTESIAN_POINT('Ctrl Pts',(-0.126657922659285,8.80032312977707E-6,
3.55565803263806));
#27674=CARTESIAN_POINT('Ctrl Pts',(-0.126658305335383,0.00043204034557634,
3.55563127527141));
#27675=CARTESIAN_POINT('Ctrl Pts',(-0.126656367352663,0.000855276509828617,
3.55560451790477));
#27676=CARTESIAN_POINT('Ctrl Pts',(-0.126652098121077,0.00127848889899514,
3.55557776053813));
#27677=CARTESIAN_POINT('Ctrl Pts',(-0.126229830197349,0.0431382506048763,
3.5529312005125));
#27678=CARTESIAN_POINT('Ctrl Pts',(-0.103000707566798,0.0847654181274417,
3.55028464048688));
#27679=CARTESIAN_POINT('Ctrl Pts',(-0.0675987137490504,0.107109477361251,
3.54763808046125));
#27680=CARTESIAN_POINT('Ctrl Pts',(-0.0321967199313031,0.12945353659506,
3.54499152043563));
#27681=CARTESIAN_POINT('Ctrl Pts',(0.0153781450736419,0.132514487540114,
3.54234496041));
#27682=CARTESIAN_POINT('Ctrl Pts',(0.0533465621421041,0.114879483210429,
3.53969840038438));
#27683=CARTESIAN_POINT('Ctrl Pts',(0.0913149792105665,0.097244478880744,
3.53705184035875));
#27684=CARTESIAN_POINT('Ctrl Pts',(0.119676948342547,0.0589135192763201,
3.53440528033313));
#27685=CARTESIAN_POINT('Ctrl Pts',(0.125448844532432,0.0174567066922002,
3.5317587203075));
#27686=CARTESIAN_POINT('Ctrl Pts',(0.131220740722318,-0.0240001058919198,
3.52911216028188));
#27687=CARTESIAN_POINT('Ctrl Pts',(0.11440256397011,-0.0685827714557354,
3.52646560025625));
#27688=CARTESIAN_POINT('Ctrl Pts',(0.0826932442631274,-0.0959262477461666,
3.52381904023063));
#27689=CARTESIAN_POINT('Ctrl Pts',(0.0509839245561443,-0.123269724036598,
3.521172480205));
#27690=CARTESIAN_POINT('Ctrl Pts',(0.00438346189438567,-0.133374011053645,
3.51852592017938));
#27691=CARTESIAN_POINT('Ctrl Pts',(-0.0357753168513136,-0.121524408044806,
3.51587936015375));
#27692=CARTESIAN_POINT('Ctrl Pts',(-0.0759340955970119,-0.109674805035968,
3.51323280012813));
#27693=CARTESIAN_POINT('Ctrl Pts',(-0.109651190426652,-0.0758713120012468,
3.5105862401025));
#27694=CARTESIAN_POINT('Ctrl Pts',(-0.121481718337573,-0.0357885021759826,
3.50793968007688));
#27695=CARTESIAN_POINT('Ctrl Pts',(-0.124881489291372,-0.0242697961962776,
3.5071791309306));
#27696=CARTESIAN_POINT('Ctrl Pts',(-0.126473800166976,-0.012232524903913,
3.50641858178433));
#27697=CARTESIAN_POINT('Ctrl Pts',(-0.126365398388193,-0.00016976464794081,
3.50565803263806));
#27698=CARTESIAN_POINT('Ctrl Pts',(-0.126245375007135,3.12536796039931E-5,
3.51934196736194));
#27699=CARTESIAN_POINT('Ctrl Pts',(-0.12620420233203,-0.0227115638743483,
3.52076771003711));
#27700=CARTESIAN_POINT('Ctrl Pts',(-0.120346328214258,-0.0454763003201931,
3.52219345271228));
#27701=CARTESIAN_POINT('Ctrl Pts',(-0.108800985171859,-0.06484981090145,
3.52361919538745));
#27702=CARTESIAN_POINT('Ctrl Pts',(-0.0873697382082225,-0.100812232138721,
3.52626575541307));
#27703=CARTESIAN_POINT('Ctrl Pts',(-0.0463410109843132,-0.125089405892421,
3.5289123154387));
#27704=CARTESIAN_POINT('Ctrl Pts',(-0.0045038827259274,-0.126577024986295,
3.53155887546432));
#27705=CARTESIAN_POINT('Ctrl Pts',(0.0373332455324584,-0.128064644080169,
3.53420543548995));
#27706=CARTESIAN_POINT('Ctrl Pts',(0.0799787748253208,-0.106762708514216,
3.53685199551558));
#27707=CARTESIAN_POINT('Ctrl Pts',(0.103913443798274,-0.0724181339568129,
3.5394985555412));
#27708=CARTESIAN_POINT('Ctrl Pts',(0.127848112771228,-0.0380735593994097,
3.54214511556683));
#27709=CARTESIAN_POINT('Ctrl Pts',(0.133071921424273,0.00931365414944368,
3.54479167559245));
#27710=CARTESIAN_POINT('Ctrl Pts',(0.117191739814205,0.0480476856196858,
3.54743823561807));
#27711=CARTESIAN_POINT('Ctrl Pts',(0.101311558204136,0.086781717089928,
3.5500847956437));
#27712=CARTESIAN_POINT('Ctrl Pts',(0.0643273863309551,0.116862566481559,
3.55273135566933));
#27713=CARTESIAN_POINT('Ctrl Pts',(0.0231710436075753,0.124520839933968,
3.55537791569495));
#27714=CARTESIAN_POINT('Ctrl Pts',(-0.0179852991158045,0.132179113386376,
3.55802447572058));
#27715=CARTESIAN_POINT('Ctrl Pts',(-0.0633138126893829,0.117414810899563,
3.5606710357462));
#27716=CARTESIAN_POINT('Ctrl Pts',(-0.0920640726196609,0.0869862082349088,
3.56331759577183));
#27717=CARTESIAN_POINT('Ctrl Pts',(-0.113878836874053,0.0638979719779231,
3.5653257196352));
#27718=CARTESIAN_POINT('Ctrl Pts',(-0.126149033113671,0.0317913564834069,
3.56733384349857));
#27719=CARTESIAN_POINT('Ctrl Pts',(-0.126440375727766,-0.00011573372396179,
3.56934196736194));
#27720=CARTESIAN_POINT('Origin',(0.,0.,3.7));
#27721=CARTESIAN_POINT('',(-0.126640903602401,4.27927297787234E-5,3.61934196736194));
#27722=CARTESIAN_POINT('',(-0.126360536148104,0.000106176725758032,3.60565803263806));
#27723=CARTESIAN_POINT('',(-0.12645,1.54856587752183E-17,3.7));
#27724=CARTESIAN_POINT('Ctrl Pts',(-0.126360536148104,0.000106176725758032,
3.60565803263806));
#27725=CARTESIAN_POINT('Ctrl Pts',(-0.126463554653562,0.0130615819764901,
3.6048439687585));
#27726=CARTESIAN_POINT('Ctrl Pts',(-0.124630630169346,0.0259885352839278,
3.60402990487894));
#27727=CARTESIAN_POINT('Ctrl Pts',(-0.120740583509641,0.0382635675762761,
3.60321584099939));
#27728=CARTESIAN_POINT('Ctrl Pts',(-0.108093858546251,0.0781702758752103,
3.60056928097376));
#27729=CARTESIAN_POINT('Ctrl Pts',(-0.0737047770896513,0.111186630609157,
3.59792272094814));
#27730=CARTESIAN_POINT('Ctrl Pts',(-0.0333162689132352,0.122198227017938,
3.59527616092251));
#27731=CARTESIAN_POINT('Ctrl Pts',(0.00707223926318085,0.133209823426719,
3.59262960089688));
#27732=CARTESIAN_POINT('Ctrl Pts',(0.0534601741594139,0.122216661510335,
3.58998304087126));
#27733=CARTESIAN_POINT('Ctrl Pts',(0.0846116648984234,0.0942510766887394,
3.58733648084563));
#27734=CARTESIAN_POINT('Ctrl Pts',(0.115763155637433,0.0662854918671437,
3.58468992082001));
#27735=CARTESIAN_POINT('Ctrl Pts',(0.131678202219219,0.0213474841403372,
3.58204336079438));
#27736=CARTESIAN_POINT('Ctrl Pts',(0.125071080316048,-0.0199904290876357,
3.57939680076876));
#27737=CARTESIAN_POINT('Ctrl Pts',(0.118463958412876,-0.0613283423156084,
3.57675024074313));
#27738=CARTESIAN_POINT('Ctrl Pts',(0.0893346680247476,-0.0990661610447472,
3.57410368071751));
#27739=CARTESIAN_POINT('Ctrl Pts',(0.0510182611448099,-0.115928737877881,
3.57145712069188));
#27740=CARTESIAN_POINT('Ctrl Pts',(0.0127018542648722,-0.132791314711016,
3.56881056066626));
#27741=CARTESIAN_POINT('Ctrl Pts',(-0.0348016691068745,-0.128778649648146,
3.56616400064063));
#27742=CARTESIAN_POINT('Ctrl Pts',(-0.069745724184294,-0.105726139172113,
3.56351744061501));
#27743=CARTESIAN_POINT('Ctrl Pts',(-0.104336486351438,-0.0829066951932904,
3.56089763795602));
#27744=CARTESIAN_POINT('Ctrl Pts',(-0.126620455001409,-0.0414304545565597,
3.55827783529704));
#27745=CARTESIAN_POINT('Ctrl Pts',(-0.126657922659285,8.80032312977707E-6,
3.55565803263806));
#27746=CARTESIAN_POINT('Ctrl Pts',(-0.126440375727766,-0.00011573372396179,
3.56934196736194));
#27747=CARTESIAN_POINT('Ctrl Pts',(-0.126533001319164,-0.0102598491305144,
3.5699804035242));
#27748=CARTESIAN_POINT('Ctrl Pts',(-0.125414835808849,-0.020383797044434,
3.57061883968645));
#27749=CARTESIAN_POINT('Ctrl Pts',(-0.123007652953296,-0.0301913583035261,
3.5712572758487));
#27750=CARTESIAN_POINT('Ctrl Pts',(-0.113028967069674,-0.0708474193348126,
3.57390383587433));
#27751=CARTESIAN_POINT('Ctrl Pts',(-0.0808995890154535,-0.10606663855489,
3.57655039589995));
#27752=CARTESIAN_POINT('Ctrl Pts',(-0.0413281018804841,-0.119726229337694,
3.57919695592558));
#27753=CARTESIAN_POINT('Ctrl Pts',(-0.00175661474551533,-0.133385820120498,
3.5818435159512));
#27754=CARTESIAN_POINT('Ctrl Pts',(0.0452569814702019,-0.125485782466029,
3.58449007597683));
#27755=CARTESIAN_POINT('Ctrl Pts',(0.0781904578005954,-0.0996425759257176,
3.58713663600245));
#27756=CARTESIAN_POINT('Ctrl Pts',(0.111123934130988,-0.0737993693854069,
3.58978319602808));
#27757=CARTESIAN_POINT('Ctrl Pts',(0.129977290576058,-0.0300129939592548,
3.5924297560537));
#27758=CARTESIAN_POINT('Ctrl Pts',(0.126119643637387,0.0116716003968688,
3.59507631607933));
#27759=CARTESIAN_POINT('Ctrl Pts',(0.122261996698715,0.0533561947529935,
3.59772287610496));
#27760=CARTESIAN_POINT('Ctrl Pts',(0.0956933463762995,0.0929390080390894,
3.60036943613058));
#27761=CARTESIAN_POINT('Ctrl Pts',(0.0585765347711879,0.112299501333378,
3.60301599615621));
#27762=CARTESIAN_POINT('Ctrl Pts',(0.0214597231660768,0.131659994627667,
3.60566255618183));
#27763=CARTESIAN_POINT('Ctrl Pts',(-0.0262052497217305,0.130798167930148,
3.60830911620746));
#27764=CARTESIAN_POINT('Ctrl Pts',(-0.0625979093128853,0.11010854389779,
3.61095567623308));
#27765=CARTESIAN_POINT('Ctrl Pts',(-0.0989905689040401,0.089418919865431,
3.61360223625871));
#27766=CARTESIAN_POINT('Ctrl Pts',(-0.124110915198542,0.048901498498232,
3.61624879628433));
#27767=CARTESIAN_POINT('Ctrl Pts',(-0.12645913501461,0.00710470077718534,
3.61889535630996));
#27768=CARTESIAN_POINT('Ctrl Pts',(-0.126591223576389,0.00475360959731907,
3.61904422666062));
#27769=CARTESIAN_POINT('Ctrl Pts',(-0.126651258400685,0.00239847031733228,
3.61919309701128));
#27770=CARTESIAN_POINT('Ctrl Pts',(-0.126640903602401,4.27927297787234E-5,
3.61934196736194));
#27771=CARTESIAN_POINT('Origin',(0.,0.,3.7));
#27772=CARTESIAN_POINT('',(-0.126313625852874,8.92012377725487E-5,3.66934196736194));
#27773=CARTESIAN_POINT('',(-0.126280524269743,-6.82698929511343E-5,3.65565803263806));
#27774=CARTESIAN_POINT('',(-0.12645,1.54856587752183E-17,3.7));
#27775=CARTESIAN_POINT('Ctrl Pts',(-0.126280524269743,-6.82698929511343E-5,
3.65565803263806));
#27776=CARTESIAN_POINT('Ctrl Pts',(-0.126155459137289,0.0254573418705088,
3.65405666224558));
#27777=CARTESIAN_POINT('Ctrl Pts',(-0.1186500792639,0.0510505822956786,
3.65245529185311));
#27778=CARTESIAN_POINT('Ctrl Pts',(-0.104270310346229,0.0719033403784211,
3.65085392146064));
#27779=CARTESIAN_POINT('Ctrl Pts',(-0.0805050891493468,0.106366370433962,
3.64820736143502));
#27780=CARTESIAN_POINT('Ctrl Pts',(-0.0379633950684185,0.127881407935326,
3.64556080140939));
#27781=CARTESIAN_POINT('Ctrl Pts',(0.00387966794034225,0.126599115215449,
3.64291424138376));
#27782=CARTESIAN_POINT('Ctrl Pts',(0.0457227309491033,0.125316822495572,
3.64026768135814));
#27783=CARTESIAN_POINT('Ctrl Pts',(0.0868671628856968,0.101237199554454,
3.63762112133251));
#27784=CARTESIAN_POINT('Ctrl Pts',(0.108477510477425,0.0653836202783246,
3.63497456130689));
#27785=CARTESIAN_POINT('Ctrl Pts',(0.130087858069152,0.0295300410021955,
3.63232800128126));
#27786=CARTESIAN_POINT('Ctrl Pts',(0.132164121316015,-0.018097494608945,
3.62968144125564));
#27787=CARTESIAN_POINT('Ctrl Pts',(0.113755810560665,-0.0556956347668708,
3.62703488123001));
#27788=CARTESIAN_POINT('Ctrl Pts',(0.0953474998053144,-0.0932937749247968,
3.62438832120439));
#27789=CARTESIAN_POINT('Ctrl Pts',(0.0564546150477511,-0.120862519629508,
3.62174176117876));
#27790=CARTESIAN_POINT('Ctrl Pts',(0.0148818767183724,-0.125781225334577,
3.61909520115314));
#27791=CARTESIAN_POINT('Ctrl Pts',(-0.0266908616110063,-0.130699931039647,
3.61644864112751));
#27792=CARTESIAN_POINT('Ctrl Pts',(-0.0709434535122003,-0.112968597745074,
3.61380208110189));
#27793=CARTESIAN_POINT('Ctrl Pts',(-0.0976175652277067,-0.0807044001658271,
3.61115552107626));
#27794=CARTESIAN_POINT('Ctrl Pts',(-0.116086901439685,-0.0583644505151555,
3.60932302493019));
#27795=CARTESIAN_POINT('Ctrl Pts',(-0.126128636638782,-0.0290570508647223,
3.60749052878412));
#27796=CARTESIAN_POINT('Ctrl Pts',(-0.126360536148104,0.000106176725758032,
3.60565803263806));
#27797=CARTESIAN_POINT('Ctrl Pts',(-0.126640903602401,4.27927297787234E-5,
3.61934196736194));
#27798=CARTESIAN_POINT('Ctrl Pts',(-0.126467174766239,-0.0394798628014113,
3.62183965703691));
#27799=CARTESIAN_POINT('Ctrl Pts',(-0.106479582237496,-0.0791540456794125,
3.62433734671187));
#27800=CARTESIAN_POINT('Ctrl Pts',(-0.0745372494842149,-0.102404041708738,
3.62683503638683));
#27801=CARTESIAN_POINT('Ctrl Pts',(-0.0406910508001211,-0.12703981239872,
3.62948159641246));
#27802=CARTESIAN_POINT('Ctrl Pts',(0.00657743990569856,-0.133235179703789,
3.63212815643808));
#27803=CARTESIAN_POINT('Ctrl Pts',(0.0456292459986054,-0.118153973308938,
3.63477471646371));
#27804=CARTESIAN_POINT('Ctrl Pts',(0.0846810520915122,-0.103072766914087,
3.63742127648934));
#27805=CARTESIAN_POINT('Ctrl Pts',(0.115516173571506,-0.0667149868193161,
3.64006783651496));
#27806=CARTESIAN_POINT('Ctrl Pts',(0.124018641769873,-0.0257248122789798,
3.64271439654059));
#27807=CARTESIAN_POINT('Ctrl Pts',(0.132521109968241,0.0152653622613568,
3.64536095656621));
#27808=CARTESIAN_POINT('Ctrl Pts',(0.11869092488498,0.0608879312472584,
3.64800751659183));
#27809=CARTESIAN_POINT('Ctrl Pts',(0.0888593883296617,0.0902574016134864,
3.65065407661746));
#27810=CARTESIAN_POINT('Ctrl Pts',(0.0590278517743432,0.119626871979714,
3.65330063664309));
#27811=CARTESIAN_POINT('Ctrl Pts',(0.0131949637469664,0.132743243726269,
3.65594719666871));
#27812=CARTESIAN_POINT('Ctrl Pts',(-0.027657500752443,0.123601990750641,
3.65859375669434));
#27813=CARTESIAN_POINT('Ctrl Pts',(-0.0685099652518527,0.114460737775013,
3.66124031671997));
#27814=CARTESIAN_POINT('Ctrl Pts',(-0.104382006223295,0.0830618600772021,
3.66388687674559));
#27815=CARTESIAN_POINT('Ctrl Pts',(-0.118851810998494,0.043779407059542,
3.66653343677121));
#27816=CARTESIAN_POINT('Ctrl Pts',(-0.123970265263591,0.0298838886116103,
3.66746961363479));
#27817=CARTESIAN_POINT('Ctrl Pts',(-0.126410714036168,0.0150019191305398,
3.66840579049837));
#27818=CARTESIAN_POINT('Ctrl Pts',(-0.126313625852874,8.92012377725487E-5,
3.66934196736194));
#27819=CARTESIAN_POINT('Origin',(0.,0.,3.7));
#27820=CARTESIAN_POINT('',(-0.126318202311182,-9.13759226411071E-5,3.71934196736194));
#27821=CARTESIAN_POINT('',(-0.126609590382811,-7.02044759900073E-5,3.70565803263806));
#27822=CARTESIAN_POINT('',(-0.12645,1.54856587752183E-17,3.7));
#27823=CARTESIAN_POINT('Ctrl Pts',(-0.126609590382811,-7.02044759900073E-5,
3.70565803263806));
#27824=CARTESIAN_POINT('Ctrl Pts',(-0.126357411318116,0.0377522139233435,
3.70326935573267));
#27825=CARTESIAN_POINT('Ctrl Pts',(-0.108290467899376,0.0757836426892297,
3.70088067882728));
#27826=CARTESIAN_POINT('Ctrl Pts',(-0.0786816086433086,0.099255188273642,
3.6984920019219));
#27827=CARTESIAN_POINT('Ctrl Pts',(-0.0458761575859702,0.125260737263231,
3.69584544189627));
#27828=CARTESIAN_POINT('Ctrl Pts',(0.00109788169852634,0.133392911300054,
3.69319888187064));
#27829=CARTESIAN_POINT('Ctrl Pts',(0.0407363279886946,0.119928893584969,
3.69055232184502));
#27830=CARTESIAN_POINT('Ctrl Pts',(0.0803747742788628,0.106464875869883,
3.68790576181939));
#27831=CARTESIAN_POINT('Ctrl Pts',(0.112677627574703,0.071404666402888,
3.68525920179377));
#27832=CARTESIAN_POINT('Ctrl Pts',(0.122857008829439,0.0307984304737455,
3.68261264176814));
#27833=CARTESIAN_POINT('Ctrl Pts',(0.133036390084175,-0.00980780545539708,
3.67996608174252));
#27834=CARTESIAN_POINT('Ctrl Pts',(0.121092299297808,-0.0559600678466875,
3.67731952171689));
#27835=CARTESIAN_POINT('Ctrl Pts',(0.0924926054626293,-0.08653037546552,
3.67467296169127));
#27836=CARTESIAN_POINT('Ctrl Pts',(0.0638929116274508,-0.117100683084353,
3.67202640166564));
#27837=CARTESIAN_POINT('Ctrl Pts',(0.0186376147434612,-0.132089035930727,
3.66937984164002));
#27838=CARTESIAN_POINT('Ctrl Pts',(-0.0225559247032424,-0.124633936707157,
3.66673328161439));
#27839=CARTESIAN_POINT('Ctrl Pts',(-0.063749464149946,-0.117178837483586,
3.66408672158877));
#27840=CARTESIAN_POINT('Ctrl Pts',(-0.100881246159364,-0.0872802861900701,
3.66144016156314));
#27841=CARTESIAN_POINT('Ctrl Pts',(-0.116952763007655,-0.0486254992384533,
3.65879360153752));
#27842=CARTESIAN_POINT('Ctrl Pts',(-0.123299788065177,-0.0333598025596003,
3.65774841190436));
#27843=CARTESIAN_POINT('Ctrl Pts',(-0.126362152343126,-0.016728441031668,
3.65670322227121));
#27844=CARTESIAN_POINT('Ctrl Pts',(-0.126280524269743,-6.82698929511343E-5,
3.65565803263806));
#27845=CARTESIAN_POINT('Ctrl Pts',(-0.126313625852874,8.92012377725487E-5,
3.66934196736194));
#27846=CARTESIAN_POINT('Ctrl Pts',(-0.126136246983132,-0.027156143714207,
3.67105235052399));
#27847=CARTESIAN_POINT('Ctrl Pts',(-0.117488868450918,-0.0545041232450019,
3.67276273368604));
#27848=CARTESIAN_POINT('Ctrl Pts',(-0.101228105076468,-0.0761266063810683,
3.67447311684809));
#27849=CARTESIAN_POINT('Ctrl Pts',(-0.0760670258002872,-0.10958413846651,
3.67711967687372));
#27850=CARTESIAN_POINT('Ctrl Pts',(-0.0326772986689716,-0.129333174299883,
3.67976623689934));
#27851=CARTESIAN_POINT('Ctrl Pts',(0.00907775247578101,-0.126332829739009,
3.68241279692497));
#27852=CARTESIAN_POINT('Ctrl Pts',(0.050832803620533,-0.123332485178135,
3.68505935695059));
#27853=CARTESIAN_POINT('Ctrl Pts',(0.0909531787787221,-0.0975827602230137,
3.68770591697622));
#27854=CARTESIAN_POINT('Ctrl Pts',(0.11107222624856,-0.0608715862708329,
3.69035247700184));
#27855=CARTESIAN_POINT('Ctrl Pts',(0.131191273718398,-0.0241604123186516,
3.69299903702747));
#27856=CARTESIAN_POINT('Ctrl Pts',(0.131308993499885,0.0235122106305895,
3.69564559705309));
#27857=CARTESIAN_POINT('Ctrl Pts',(0.111371494820412,0.0603222977018694,
3.69829215707872));
#27858=CARTESIAN_POINT('Ctrl Pts',(0.0914339961409399,0.097132384773149,
3.70093871710434));
#27859=CARTESIAN_POINT('Ctrl Pts',(0.0514412790005074,0.123079935966467,
3.70358527712997));
#27860=CARTESIAN_POINT('Ctrl Pts',(0.00970155469863815,0.126286457292336,
3.70623183715559));
#27861=CARTESIAN_POINT('Ctrl Pts',(-0.0320381696032317,0.129492978618205,
3.70887839718122));
#27862=CARTESIAN_POINT('Ctrl Pts',(-0.0755249010665388,0.109958470076624,
3.71152495720684));
#27863=CARTESIAN_POINT('Ctrl Pts',(-0.100850908347825,0.0766256076274997,
3.71417151723247));
#27864=CARTESIAN_POINT('Ctrl Pts',(-0.117343620441844,0.0549186998809637,
3.71589500060896));
#27865=CARTESIAN_POINT('Ctrl Pts',(-0.126134681028771,0.0273601470071565,
3.71761848398545));
#27866=CARTESIAN_POINT('Ctrl Pts',(-0.126318202311182,-9.13759226411071E-5,
3.71934196736194));
#27867=CARTESIAN_POINT('Origin',(0.,0.,3.7));
#27868=CARTESIAN_POINT('',(-0.126643738265873,-3.92119282522094E-5,3.76934196736194));
#27869=CARTESIAN_POINT('',(-0.126492921331233,0.000111898061355794,3.75565803263806));
#27870=CARTESIAN_POINT('',(-0.12645,1.54856587752183E-17,3.7));
#27871=CARTESIAN_POINT('Ctrl Pts',(-0.126492921331233,0.000111898061355794,
3.75565803263806));
#27872=CARTESIAN_POINT('Ctrl Pts',(-0.12657025228906,0.00851493641555574,
3.75512860924538));
#27873=CARTESIAN_POINT('Ctrl Pts',(-0.125804504023154,0.0169039539351017,
3.7545991858527));
#27874=CARTESIAN_POINT('Ctrl Pts',(-0.12414416907011,0.0251120135156184,
3.75406976246003));
#27875=CARTESIAN_POINT('Ctrl Pts',(-0.115844240928182,0.06614367678216,
3.7514232024344));
#27876=CARTESIAN_POINT('Ctrl Pts',(-0.0851890554053168,0.102653294996741,
3.74877664240878));
#27877=CARTESIAN_POINT('Ctrl Pts',(-0.0462122079706087,0.117927179951992,
3.74613008238315));
#27878=CARTESIAN_POINT('Ctrl Pts',(-0.00723536053590029,0.133201064907244,
3.74348352235752));
#27879=CARTESIAN_POINT('Ctrl Pts',(0.0400631488106516,0.127239216603166,
3.7408369623319));
#27880=CARTESIAN_POINT('Ctrl Pts',(0.0740306001411793,0.102770901424588,
3.73819040230627));
#27881=CARTESIAN_POINT('Ctrl Pts',(0.107998051471707,0.0783025862460102,
3.73554384228065));
#27882=CARTESIAN_POINT('Ctrl Pts',(0.12863444478621,0.0353278041929325,
3.73289728225502));
#27883=CARTESIAN_POINT('Ctrl Pts',(0.126492673803057,-0.00648007801438488,
3.7302507222294));
#27884=CARTESIAN_POINT('Ctrl Pts',(0.124350902819903,-0.0482879602217022,
3.72760416220377));
#27885=CARTESIAN_POINT('Ctrl Pts',(0.0994309675390923,-0.0889289425832592,
3.72495760217815));
#27886=CARTESIAN_POINT('Ctrl Pts',(0.063140931062625,-0.109798045345167,
3.72231104215252));
#27887=CARTESIAN_POINT('Ctrl Pts',(0.0268508945861577,-0.130667148107075,
3.7196644821269));
#27888=CARTESIAN_POINT('Ctrl Pts',(-0.020809243085966,-0.131764371269333,
3.71701792210127));
#27889=CARTESIAN_POINT('Ctrl Pts',(-0.0580212126891809,-0.112587418545307,
3.71437136207565));
#27890=CARTESIAN_POINT('Ctrl Pts',(-0.0952331822923957,-0.0934104658212808,
3.71172480205002));
#27891=CARTESIAN_POINT('Ctrl Pts',(-0.121996983826702,-0.0539593372109697,
3.7090782420244));
#27892=CARTESIAN_POINT('Ctrl Pts',(-0.126060453178764,-0.0122943109346363,
3.70643168199877));
#27893=CARTESIAN_POINT('Ctrl Pts',(-0.126456401181211,-0.00823443438662399,
3.70617379887853));
#27894=CARTESIAN_POINT('Ctrl Pts',(-0.126636815799491,-0.0041535374917583,
3.70591591575829));
#27895=CARTESIAN_POINT('Ctrl Pts',(-0.126609590382811,-7.02044759900073E-5,
3.70565803263806));
#27896=CARTESIAN_POINT('Ctrl Pts',(-0.126318202311182,-9.13759226411071E-5,
3.71934196736194));
#27897=CARTESIAN_POINT('Ctrl Pts',(-0.126416494068865,-0.0147940763636936,
3.72026504401107));
#27898=CARTESIAN_POINT('Ctrl Pts',(-0.12404567634908,-0.0294660748073717,
3.72118812066021));
#27899=CARTESIAN_POINT('Ctrl Pts',(-0.119066572492589,-0.0431919063448052,
3.72211119730934));
#27900=CARTESIAN_POINT('Ctrl Pts',(-0.104790946256804,-0.0825453415113195,
3.72475775733497));
#27901=CARTESIAN_POINT('Ctrl Pts',(-0.0690744106859675,-0.11412099548768,
3.7274043173606));
#27902=CARTESIAN_POINT('Ctrl Pts',(-0.0282675897675097,-0.123463892809314,
3.73005087738622));
#27903=CARTESIAN_POINT('Ctrl Pts',(0.0125392311509478,-0.132806790130948,
3.73269743741185));
#27904=CARTESIAN_POINT('Ctrl Pts',(0.0584363374170267,-0.119916930797855,
3.73534399743747));
#27905=CARTESIAN_POINT('Ctrl Pts',(0.0884125555029259,-0.0906951458916328,
3.7379905574631));
#27906=CARTESIAN_POINT('Ctrl Pts',(0.118388773588825,-0.0614733609854108,
3.74063711748872));
#27907=CARTESIAN_POINT('Ctrl Pts',(0.132444103494545,-0.0159196505060593,
3.74328367751435));
#27908=CARTESIAN_POINT('Ctrl Pts',(0.124144174958903,0.0251120147068241,
3.74593023753997));
#27909=CARTESIAN_POINT('Ctrl Pts',(0.115844246423262,0.0661436799197074,
3.7485767975656));
#27910=CARTESIAN_POINT('Ctrl Pts',(0.0851890594462595,0.102653299866123,
3.75122335759122));
#27911=CARTESIAN_POINT('Ctrl Pts',(0.0462122101626772,0.117927185545889,
3.75386991761685));
#27912=CARTESIAN_POINT('Ctrl Pts',(0.00723536087909469,0.133201071225655,
3.75651647764247));
#27913=CARTESIAN_POINT('Ctrl Pts',(-0.0400631507110678,0.127239222638772,
3.7591630376681));
#27914=CARTESIAN_POINT('Ctrl Pts',(-0.0740306036528435,0.102770906299531,
3.76180959769372));
#27915=CARTESIAN_POINT('Ctrl Pts',(-0.106255505634774,0.0795578294448588,
3.76432038758313));
#27916=CARTESIAN_POINT('Ctrl Pts',(-0.12648204772981,0.0396883664632768,
3.76683117747254));
#27917=CARTESIAN_POINT('Ctrl Pts',(-0.126643738265873,-3.92119282522094E-5,
3.76934196736194));
#27918=CARTESIAN_POINT('Origin',(0.,0.,3.7));
#27919=CARTESIAN_POINT('',(-0.12643411897368,0.000115681837355761,3.81934196736194));
#27920=CARTESIAN_POINT('',(-0.126243465328102,1.71616150689059E-6,3.80565803263806));
#27921=CARTESIAN_POINT('',(-0.12645,1.54856587752183E-17,3.7));
#27922=CARTESIAN_POINT('Ctrl Pts',(-0.126243465328102,1.71616150689059E-6,
3.80565803263806));
#27923=CARTESIAN_POINT('Ctrl Pts',(-0.126246007062352,0.0210055997219054,
3.80434130273247));
#27924=CARTESIAN_POINT('Ctrl Pts',(-0.121290894068088,0.0420083553470164,
3.80302457282688));
#27925=CARTESIAN_POINT('Ctrl Pts',(-0.111371489537494,0.0603222948404575,
3.80170784292128));
#27926=CARTESIAN_POINT('Ctrl Pts',(-0.0914339918037617,0.0971323801656441,
3.79906128289566));
#27927=CARTESIAN_POINT('Ctrl Pts',(-0.0514412765603963,0.123079930128149,
3.79641472287003));
#27928=CARTESIAN_POINT('Ctrl Pts',(-0.00970155423845781,0.126286451301922,
3.79376816284441));
#27929=CARTESIAN_POINT('Ctrl Pts',(0.0320381680834807,0.129492972475696,
3.79112160281878));
#27930=CARTESIAN_POINT('Ctrl Pts',(0.0755248974839926,0.109958464860738,
3.78847504279316));
#27931=CARTESIAN_POINT('Ctrl Pts',(0.10085090356394,0.0766256039927644,
3.78582848276753));
#27932=CARTESIAN_POINT('Ctrl Pts',(0.126176909643887,0.0432927431247909,
3.78318192274191));
#27933=CARTESIAN_POINT('Ctrl Pts',(0.13334219240327,-0.00383847099619805,
3.78053536271628));
#27934=CARTESIAN_POINT('Ctrl Pts',(0.119066566844655,-0.0431919042959778,
3.77788880269065));
#27935=CARTESIAN_POINT('Ctrl Pts',(0.10479094128604,-0.0825453375957573,
3.77524224266503));
#27936=CARTESIAN_POINT('Ctrl Pts',(0.0690744074094266,-0.114120990074327,
3.7725956826394));
#27937=CARTESIAN_POINT('Ctrl Pts',(0.0282675884266474,-0.123463886952785,
3.76994912261378));
#27938=CARTESIAN_POINT('Ctrl Pts',(-0.0125392305561318,-0.132806783831242,
3.76730256258815));
#27939=CARTESIAN_POINT('Ctrl Pts',(-0.0584363346450773,-0.119916925109586,
3.76465600256253));
#27940=CARTESIAN_POINT('Ctrl Pts',(-0.088412551309054,-0.0906951415895065,
3.7620094425369));
#27941=CARTESIAN_POINT('Ctrl Pts',(-0.112392263011044,-0.0673189446502994,
3.75989230590395));
#27942=CARTESIAN_POINT('Ctrl Pts',(-0.126183678849807,-0.0334914156074963,
3.75777516927101));
#27943=CARTESIAN_POINT('Ctrl Pts',(-0.126492921331233,0.000111898061355794,
3.75565803263806));
#27944=CARTESIAN_POINT('Ctrl Pts',(-0.126643738265873,-3.92119282522094E-5,
3.76934196736194));
#27945=CARTESIAN_POINT('Ctrl Pts',(-0.12665248162835,-0.00218746764357669,
3.76947773749816));
#27946=CARTESIAN_POINT('Ctrl Pts',(-0.126602553960315,-0.00433530847842783,
3.76961350763438));
#27947=CARTESIAN_POINT('Ctrl Pts',(-0.126492679803253,-0.0064800783217853,
3.7697492777706));
#27948=CARTESIAN_POINT('Ctrl Pts',(-0.124350908718499,-0.0482879625122638,
3.77239583779623));
#27949=CARTESIAN_POINT('Ctrl Pts',(-0.0994309722556023,-0.0889289468016232,
3.77504239782185));
#27950=CARTESIAN_POINT('Ctrl Pts',(-0.0631409340577098,-0.109798050553457,
3.77768895784748));
#27951=CARTESIAN_POINT('Ctrl Pts',(-0.0268508958598173,-0.130667154305292,
3.7803355178731));
#27952=CARTESIAN_POINT('Ctrl Pts',(0.0208092440730706,-0.131764377519601,
3.78298207789873));
#27953=CARTESIAN_POINT('Ctrl Pts',(0.0580212154414384,-0.112587423885904,
3.78562863792435));
#27954=CARTESIAN_POINT('Ctrl Pts',(0.0952331868098064,-0.0934104702522078,
3.78827519794998));
#27955=CARTESIAN_POINT('Ctrl Pts',(0.121996989613654,-0.0539593397705055,
3.7909217579756));
#27956=CARTESIAN_POINT('Ctrl Pts',(0.126060459158462,-0.0122943115177929,
3.79356831800123));
#27957=CARTESIAN_POINT('Ctrl Pts',(0.130123928703269,0.0293707167349194,
3.79621487802685));
#27958=CARTESIAN_POINT('Ctrl Pts',(0.111487064989038,0.073249642758642,
3.79886143805248));
#27959=CARTESIAN_POINT('Ctrl Pts',(0.0786816123755665,0.0992551929818185,
3.8015079980781));
#27960=CARTESIAN_POINT('Ctrl Pts',(0.0458761597620954,0.125260743204995,
3.80415455810373));
#27961=CARTESIAN_POINT('Ctrl Pts',(-0.00109788175061491,0.133392917627625,
3.80680111812935));
#27962=CARTESIAN_POINT('Ctrl Pts',(-0.0407363299210399,0.119928899273839,
3.80944767815498));
#27963=CARTESIAN_POINT('Ctrl Pts',(-0.0803747780914649,0.106464880920053,
3.81209423818061));
#27964=CARTESIAN_POINT('Ctrl Pts',(-0.112677632919605,0.071404669789851,
3.81474079820623));
#27965=CARTESIAN_POINT('Ctrl Pts',(-0.122857014657189,0.030798431934596,
3.81738735823185));
#27966=CARTESIAN_POINT('Ctrl Pts',(-0.125362998814015,0.0208018927186779,
3.81803889460855));
#27967=CARTESIAN_POINT('Ctrl Pts',(-0.126528173261855,0.0104692323861157,
3.81869043098525));
#27968=CARTESIAN_POINT('Ctrl Pts',(-0.12643411897368,0.000115681837355761,
3.81934196736194));
#27969=CARTESIAN_POINT('Origin',(0.,0.,3.7));
#27970=CARTESIAN_POINT('',(-0.126249985800877,-2.99474503126992E-5,3.86934196736194));
#27971=CARTESIAN_POINT('',(-0.126486618721746,-0.000112766438119152,3.85565803263806));
#27972=CARTESIAN_POINT('',(-0.12645,1.54856587752183E-17,3.7));
#27973=CARTESIAN_POINT('Ctrl Pts',(-0.126486618721746,-0.000112766438119152,
3.85565803263806));
#27974=CARTESIAN_POINT('Ctrl Pts',(-0.126178545401481,0.0332869000256312,
3.85355399621955));
#27975=CARTESIAN_POINT('Ctrl Pts',(-0.112575693492532,0.0669084342579941,
3.85144995980104));
#27976=CARTESIAN_POINT('Ctrl Pts',(-0.0888593841145145,0.0902573973319142,
3.84934592338254));
#27977=CARTESIAN_POINT('Ctrl Pts',(-0.0590278489741825,0.119626866304839,
3.84669936335691));
#27978=CARTESIAN_POINT('Ctrl Pts',(-0.0131949631210826,0.13274323742959,
3.84405280333129));
#27979=CARTESIAN_POINT('Ctrl Pts',(0.0276574994404428,0.123601984887668,
3.84140624330566));
#27980=CARTESIAN_POINT('Ctrl Pts',(0.0685099620019675,0.114460732345747,
3.83875968328004));
#27981=CARTESIAN_POINT('Ctrl Pts',(0.104382001271918,0.0830618561371527,
3.83611312325441));
#27982=CARTESIAN_POINT('Ctrl Pts',(0.118851805360766,0.0437794049828168,
3.83346656322878));
#27983=CARTESIAN_POINT('Ctrl Pts',(0.133321609449615,0.00449695382848087,
3.83082000320316));
#27984=CARTESIAN_POINT('Ctrl Pts',(0.126389178357361,-0.0426690722715969,
3.82817344317753));
#27985=CARTESIAN_POINT('Ctrl Pts',(0.101228100274691,-0.0761266027699533,
3.82552688315191));
#27986=CARTESIAN_POINT('Ctrl Pts',(0.0760670221920212,-0.10958413326831,
3.82288032312628));
#27987=CARTESIAN_POINT('Ctrl Pts',(0.0326772971189339,-0.129333168164945,
3.82023376310066));
#27988=CARTESIAN_POINT('Ctrl Pts',(-0.0090777520451555,-0.12633282374641,
3.81758720307503));
#27989=CARTESIAN_POINT('Ctrl Pts',(-0.0508328012092449,-0.123332479327876,
3.81494064304941));
#27990=CARTESIAN_POINT('Ctrl Pts',(-0.0909531744643365,-0.097582755594171,
3.81229408302378));
#27991=CARTESIAN_POINT('Ctrl Pts',(-0.111072220979832,-0.0608715833833843,
3.80964752299816));
#27992=CARTESIAN_POINT('Ctrl Pts',(-0.121181537898249,-0.0424251389139816,
3.80831769287812));
#27993=CARTESIAN_POINT('Ctrl Pts',(-0.126240898306005,-0.021211136130883,
3.80698786275809));
#27994=CARTESIAN_POINT('Ctrl Pts',(-0.126243465328102,1.71616150689059E-6,
3.80565803263806));
#27995=CARTESIAN_POINT('Ctrl Pts',(-0.12643411897368,0.000115681837355761,
3.81934196736194));
#27996=CARTESIAN_POINT('Ctrl Pts',(-0.126146121962456,-0.0315871960586303,
3.82133699101087));
#27997=CARTESIAN_POINT('Ctrl Pts',(-0.114051564760291,-0.0634859411452914,
3.8233320146598));
#27998=CARTESIAN_POINT('Ctrl Pts',(-0.0924926098500027,-0.0865303795699984,
3.82532703830873));
#27999=CARTESIAN_POINT('Ctrl Pts',(-0.0638929146582029,-0.117100688639029,
3.82797359833436));
#28000=CARTESIAN_POINT('Ctrl Pts',(-0.018637615627574,-0.132089042196783,
3.83062015835998));
#28001=CARTESIAN_POINT('Ctrl Pts',(0.0225559257731756,-0.124633942619396,
3.83326671838561));
#28002=CARTESIAN_POINT('Ctrl Pts',(0.0637494671739252,-0.117178843042008,
3.83591327841123));
#28003=CARTESIAN_POINT('Ctrl Pts',(0.100881250944795,-0.0872802903294789,
3.83855983843686));
#28004=CARTESIAN_POINT('Ctrl Pts',(0.116952768555385,-0.048625501544595,
3.84120639846248));
#28005=CARTESIAN_POINT('Ctrl Pts',(0.133024286165975,-0.00997071275971127,
3.84385295848811));
#28006=CARTESIAN_POINT('Ctrl Pts',(0.128035537616284,0.0374403120975275,
3.84649951851373));
#28007=CARTESIAN_POINT('Ctrl Pts',(0.10427031529219,0.0719033437884345,
3.84914607853936));
#28008=CARTESIAN_POINT('Ctrl Pts',(0.080505092968096,0.106366375479342,
3.85179263856498));
#28009=CARTESIAN_POINT('Ctrl Pts',(0.037963396869598,0.127881414003918,
3.85443919859061));
#28010=CARTESIAN_POINT('Ctrl Pts',(-0.003879668124188,0.126599121222081,
3.85708575861623));
#28011=CARTESIAN_POINT('Ctrl Pts',(-0.0457227331179738,0.125316828440245,
3.85973231864186));
#28012=CARTESIAN_POINT('Ctrl Pts',(-0.0868671670070475,0.101237204351996,
3.86237887866749));
#28013=CARTESIAN_POINT('Ctrl Pts',(-0.108477515623481,0.0653836233772192,
3.86502543869311));
#28014=CARTESIAN_POINT('Ctrl Pts',(-0.120226312608128,0.0458912749879413,
3.86646428158272));
#28015=CARTESIAN_POINT('Ctrl Pts',(-0.126201381437229,0.0229188749131541,
3.86790312447233));
#28016=CARTESIAN_POINT('Ctrl Pts',(-0.126249985800877,-2.99474503126992E-5,
3.86934196736194));
#28017=CARTESIAN_POINT('Origin',(0.,0.,3.7));
#28018=CARTESIAN_POINT('',(-0.126543984365092,-0.000100563349596846,3.91934196736194));
#28019=CARTESIAN_POINT('',(-0.126614009842867,6.71750503076223E-5,3.90565803263806));
#28020=CARTESIAN_POINT('',(-0.12645,1.54856587752183E-17,3.7));
#28021=CARTESIAN_POINT('Ctrl Pts',(-0.126614009842867,6.71750503076223E-5,
3.90565803263806));
#28022=CARTESIAN_POINT('Ctrl Pts',(-0.126638949568151,0.00394272317787337,
3.90541324973226));
#28023=CARTESIAN_POINT('Ctrl Pts',(-0.126476435154099,0.00781615144459198,
3.90516846682647));
#28024=CARTESIAN_POINT('Ctrl Pts',(-0.126119637661472,0.0116715998582211,
3.90492368392067));
#28025=CARTESIAN_POINT('Ctrl Pts',(-0.122261990910541,0.0533561922490439,
3.90227712389504));
#28026=CARTESIAN_POINT('Ctrl Pts',(-0.0956933418361204,0.0929390036289487,
3.89963056386942));
#28027=CARTESIAN_POINT('Ctrl Pts',(-0.0585765319889427,0.112299495998321,
3.89698400384379));
#28028=CARTESIAN_POINT('Ctrl Pts',(-0.0214597221417651,0.131659988367694,
3.89433744381817));
#28029=CARTESIAN_POINT('Ctrl Pts',(0.0262052484781696,0.130798161726534,
3.89169088379254));
#28030=CARTESIAN_POINT('Ctrl Pts',(0.0625979063415064,0.110108538679153,
3.88904432376692));
#28031=CARTESIAN_POINT('Ctrl Pts',(0.0989905642048431,0.089418915631772,
3.88639776374129));
#28032=CARTESIAN_POINT('Ctrl Pts',(0.124110909311582,0.04890149617817,3.88375120371567));
#28033=CARTESIAN_POINT('Ctrl Pts',(0.12645912901712,0.0071047004378325,
3.88110464369004));
#28034=CARTESIAN_POINT('Ctrl Pts',(0.128807348722658,-0.0346920953025048,
3.87845808366442));
#28035=CARTESIAN_POINT('Ctrl Pts',(0.108383443026996,-0.0777682673295779,
3.87581152363879));
#28036=CARTESIAN_POINT('Ctrl Pts',(0.0745372459479278,-0.102404036849921,
3.87316496361316));
#28037=CARTESIAN_POINT('Ctrl Pts',(0.0406910488688595,-0.127039806370264,
3.87051840358754));
#28038=CARTESIAN_POINT('Ctrl Pts',(-0.00657743959361464,-0.133235173383876,
3.86787184356191));
#28039=CARTESIAN_POINT('Ctrl Pts',(-0.0456292438338329,-0.118153967704968,
3.86522528353629));
#28040=CARTESIAN_POINT('Ctrl Pts',(-0.0846810480740508,-0.10307276202606,
3.86257872351066));
#28041=CARTESIAN_POINT('Ctrl Pts',(-0.115516168092013,-0.0667149836546316,
3.85993216348504));
#28042=CARTESIAN_POINT('Ctrl Pts',(-0.124018635887212,-0.0257248110583692,
3.85728560345941));
#28043=CARTESIAN_POINT('Ctrl Pts',(-0.125761573683066,-0.0173221539948553,
3.85674307985229));
#28044=CARTESIAN_POINT('Ctrl Pts',(-0.126566055107683,-0.00872483577640936,
3.85620055624518));
#28045=CARTESIAN_POINT('Ctrl Pts',(-0.126486618721746,-0.000112766438119152,
3.85565803263806));
#28046=CARTESIAN_POINT('Ctrl Pts',(-0.126249985800877,-2.99474503126992E-5,
3.86934196736194));
#28047=CARTESIAN_POINT('Ctrl Pts',(-0.126290782696275,-0.01929242997697,
3.87054968449796));
#28048=CARTESIAN_POINT('Ctrl Pts',(-0.12215616704665,-0.0385383011374065,
3.87175740163397));
#28049=CARTESIAN_POINT('Ctrl Pts',(-0.113755815955893,-0.0556956374040618,
3.87296511876998));
#28050=CARTESIAN_POINT('Ctrl Pts',(-0.0953475043280787,-0.0932937793492606,
3.87561167879561));
#28051=CARTESIAN_POINT('Ctrl Pts',(-0.0564546177286578,-0.120862525378353,
3.87825823882124));
#28052=CARTESIAN_POINT('Ctrl Pts',(-0.0148818774258165,-0.125781231309797,
3.88090479884686));
#28053=CARTESIAN_POINT('Ctrl Pts',(0.0266908628770249,-0.13069993724124,
3.88355135887249));
#28054=CARTESIAN_POINT('Ctrl Pts',(0.0709434568832867,-0.112968603075036,
3.88619791889811));
#28055=CARTESIAN_POINT('Ctrl Pts',(0.0976175698612337,-0.0807044039779288,
3.88884447892374));
#28056=CARTESIAN_POINT('Ctrl Pts',(0.124291682839181,-0.0484402048808214,
3.89149103894936));
#28057=CARTESIAN_POINT('Ctrl Pts',(0.133387314788813,-0.00164314085281106,
3.89413759897499));
#28058=CARTESIAN_POINT('Ctrl Pts',(0.120740589231085,0.0382635693618544,
3.89678415900061));
#28059=CARTESIAN_POINT('Ctrl Pts',(0.108093863673357,0.0781702795765198,
3.89943071902624));
#28060=CARTESIAN_POINT('Ctrl Pts',(0.0737047806082696,0.11118663597784,
3.90207727905187));
#28061=CARTESIAN_POINT('Ctrl Pts',(0.0333162705051194,0.122198232868137,
3.90472383907749));
#28062=CARTESIAN_POINT('Ctrl Pts',(-0.00707223959803082,0.133209829758434,
3.90737039910312));
#28063=CARTESIAN_POINT('Ctrl Pts',(-0.0534601767392434,0.122216667137707,
3.91001695912874));
#28064=CARTESIAN_POINT('Ctrl Pts',(-0.0846116689345932,0.0942510810621984,
3.91266351915437));
#28065=CARTESIAN_POINT('Ctrl Pts',(-0.110814692885301,0.0707278765512593,
3.91488966855689));
#28066=CARTESIAN_POINT('Ctrl Pts',(-0.126237468513852,0.0351961661111841,
3.91711581795942));
#28067=CARTESIAN_POINT('Ctrl Pts',(-0.126543984365092,-0.000100563349596846,
3.91934196736194));
#28068=CARTESIAN_POINT('Origin',(0.,0.,3.7));
#28069=CARTESIAN_POINT('',(-0.126567406925801,8.9117089303592E-5,3.96934196736194));
#28070=CARTESIAN_POINT('',(-0.126283770505697,7.06948412972308E-5,3.95565803263806));
#28071=CARTESIAN_POINT('',(-0.12645,1.54856587752183E-17,3.7));
#28072=CARTESIAN_POINT('',(0.0958116152722338,0.0825211298936549,4.));
#28073=CARTESIAN_POINT('Ctrl Pts',(-0.126567406925801,8.9117089303592E-5,
3.96934196736194));
#28074=CARTESIAN_POINT('Ctrl Pts',(-0.126271512495954,-0.03602989561222,
3.97162163149775));
#28075=CARTESIAN_POINT('Ctrl Pts',(-0.11000667585855,-0.0723734458913716,
3.97390129563356));
#28076=CARTESIAN_POINT('Ctrl Pts',(-0.0826932529987204,-0.0959262598695684,
3.97618095976937));
#28077=CARTESIAN_POINT('Ctrl Pts',(-0.0509839270641226,-0.123269733404333,
3.978827519795));
#28078=CARTESIAN_POINT('Ctrl Pts',(-0.0043834430999392,-0.133373998977298,
3.98147407982063));
#28079=CARTESIAN_POINT('Ctrl Pts',(0.0357753280219188,-0.121524403040669,
3.98412063984625));
#28080=CARTESIAN_POINT('Ctrl Pts',(0.0759340991437768,-0.109674807104039,
3.98676719987188));
#28081=CARTESIAN_POINT('Ctrl Pts',(0.109651157423309,-0.0758713496578151,
3.9894137598975));
#28082=CARTESIAN_POINT('Ctrl Pts',(0.121481684447537,-0.0357885393155276,
3.99206031992312));
#28083=CARTESIAN_POINT('Ctrl Pts',(0.133312211471764,0.00429427102675994,
3.99470687994875));
#28084=CARTESIAN_POINT('Ctrl Pts',(0.123256207240687,0.0506564342651108,
3.99735343997437));
#28085=CARTESIAN_POINT('Ctrl Pts',(0.095811615272233,0.0825211298936557,
4.));
#28086=CARTESIAN_POINT('',(-0.0959939867336434,0.082660026050108,4.));
#28087=CARTESIAN_POINT('Origin',(0.,0.,4.));
#28088=CARTESIAN_POINT('Ctrl Pts',(-0.095994151316856,0.0826601513985344,
4.));
#28089=CARTESIAN_POINT('Ctrl Pts',(-0.0693049200029063,0.113544200686508,
3.9974200549221));
#28090=CARTESIAN_POINT('Ctrl Pts',(-0.0262885035315151,0.130447365396717,
3.9948401098442));
#28091=CARTESIAN_POINT('Ctrl Pts',(0.0142676559974625,0.125842964228272,
3.9922601647663));
#28092=CARTESIAN_POINT('Ctrl Pts',(0.0558709876039151,0.121119676054917,
3.98961360474068));
#28093=CARTESIAN_POINT('Ctrl Pts',(0.0948853729157606,0.0937638197023474,
3.98696704471505));
#28094=CARTESIAN_POINT('Ctrl Pts',(0.113475682659087,0.0562620533584955,
3.98432048468943));
#28095=CARTESIAN_POINT('Ctrl Pts',(0.132065992402412,0.0187602870146438,
3.9816739246638));
#28096=CARTESIAN_POINT('Ctrl Pts',(0.130232226577219,-0.0288873893204904,
3.97902736463818));
#28097=CARTESIAN_POINT('Ctrl Pts',(0.108800980591427,-0.0648498109281795,
3.97638080461255));
#28098=CARTESIAN_POINT('Ctrl Pts',(0.0873697346056348,-0.100812232535869,
3.97373424458693));
#28099=CARTESIAN_POINT('Ctrl Pts',(0.046341008459244,-0.125089399416112,
3.9710876845613));
#28100=CARTESIAN_POINT('Ctrl Pts',(0.00450388209284308,-0.126577017215687,
3.96844112453568));
#28101=CARTESIAN_POINT('Ctrl Pts',(-0.0373332442735578,-0.128064635015261,
3.96579456451005));
#28102=CARTESIAN_POINT('Ctrl Pts',(-0.0799787708599689,-0.106762703734165,
3.96314800448442));
#28103=CARTESIAN_POINT('Ctrl Pts',(-0.103913438592044,-0.0724181315163075,
3.9605014444588));
#28104=CARTESIAN_POINT('Ctrl Pts',(-0.118514209844363,-0.0514670471592998,
3.95888697385188));
#28105=CARTESIAN_POINT('Ctrl Pts',(-0.126152075437054,-0.0256623813017284,
3.95727250324497));
#28106=CARTESIAN_POINT('Ctrl Pts',(-0.126283770505697,7.06948412972308E-5,
3.95565803263806));
#28107=CARTESIAN_POINT('Origin',(0.,0.,4.11042117235887));
#28108=CARTESIAN_POINT('',(-0.154553716617854,1.07385516829317E-5,3.53957882764113));
#28109=CARTESIAN_POINT('',(-0.154050307343621,3.81371511608408E-5,3.53542117235887));
#28110=CARTESIAN_POINT('',(-0.1543,7.47606542906876E-15,4.11042117235887));
#28111=CARTESIAN_POINT('',(0.0398513841857357,-0.149064942821848,3.5));
#28112=CARTESIAN_POINT('Ctrl Pts',(-0.154050307343621,3.81371511608431E-5,
3.53542117235887));
#28113=CARTESIAN_POINT('Ctrl Pts',(-0.154093326879583,0.0238011172149125,
3.53420035500841));
#28114=CARTESIAN_POINT('Ctrl Pts',(-0.137743852801688,0.0990167675561842,
3.53033297763233));
#28115=CARTESIAN_POINT('Ctrl Pts',(-0.0205691901156568,0.181176596665036,
3.52381904023063));
#28116=CARTESIAN_POINT('Ctrl Pts',(0.141207069227503,0.115615351338242,
3.51587936015375));
#28117=CARTESIAN_POINT('Ctrl Pts',(0.173454096992073,-0.0561631599472297,
3.50793968007688));
#28118=CARTESIAN_POINT('Ctrl Pts',(0.089426887306191,-0.135811307301286,
3.50264656002563));
#28119=CARTESIAN_POINT('Ctrl Pts',(0.0398513841857336,-0.149064942821849,
3.5));
#28120=CARTESIAN_POINT('',(-0.0398513841857265,-0.149064942821851,3.5));
#28121=CARTESIAN_POINT('Origin',(0.,0.,3.5));
#28122=CARTESIAN_POINT('Ctrl Pts',(-0.154553716617854,1.07385516829459E-5,
3.53957882764113));
#28123=CARTESIAN_POINT('Ctrl Pts',(-0.154554183576509,0.000527195138975443,
3.53955207027449));
#28124=CARTESIAN_POINT('Ctrl Pts',(-0.154317915988944,0.0521256879879336,
3.53687875288222));
#28125=CARTESIAN_POINT('Ctrl Pts',(-0.0973408901199132,0.154229940417525,
3.53155887546432));
#28126=CARTESIAN_POINT('Ctrl Pts',(0.0768181056158631,0.16543527210962,
3.52361919538745));
#28127=CARTESIAN_POINT('Ctrl Pts',(0.180643771975638,0.0251157687415861,
3.51567951531057));
#28128=CARTESIAN_POINT('Ctrl Pts',(0.119593430082514,-0.13672026231454,
3.50780645018142));
#28129=CARTESIAN_POINT('Ctrl Pts',(0.00819996357198913,-0.162114976519676,
3.5025799450779));
#28130=CARTESIAN_POINT('Ctrl Pts',(-0.0399398165374138,-0.14933059314829,
3.5));
#28131=CARTESIAN_POINT('Origin',(0.,0.,4.11042117235887));
#28132=CARTESIAN_POINT('',(-0.15419083216807,0.000129561635314926,3.58957882764113));
#28133=CARTESIAN_POINT('',(-0.154288256028425,-0.000141223516069758,3.58542117235887));
#28134=CARTESIAN_POINT('',(-0.1543,7.47606542906876E-15,4.11042117235887));
#28135=CARTESIAN_POINT('Ctrl Pts',(-0.154288256028425,-0.000141223516069763,
3.58542117235887));
#28136=CARTESIAN_POINT('Ctrl Pts',(-0.153932746614783,0.0387932487575316,
3.5834130484955));
#28137=CARTESIAN_POINT('Ctrl Pts',(-0.119227247372343,0.129604846059009,
3.57875836460651));
#28138=CARTESIAN_POINT('Ctrl Pts',(0.0333654249967142,0.179306991453011,
3.57145712069188));
#28139=CARTESIAN_POINT('Ctrl Pts',(0.16875469474836,0.0691889591605158,
3.56351744061501));
#28140=CARTESIAN_POINT('Ctrl Pts',(0.149631713131164,-0.104283094234219,
3.55557776053813));
#28141=CARTESIAN_POINT('Ctrl Pts',(-0.00648228852693025,-0.182263845309582,
3.54763808046125));
#28142=CARTESIAN_POINT('Ctrl Pts',(-0.133583343879226,-0.107056676726779,
3.54091921773484));
#28143=CARTESIAN_POINT('Ctrl Pts',(-0.154000066586259,-0.0277136758071254,
3.53684691503404));
#28144=CARTESIAN_POINT('Ctrl Pts',(-0.154050307343621,3.81371511608431E-5,
3.53542117235887));
#28145=CARTESIAN_POINT('Ctrl Pts',(-0.15419083216807,0.000129561635314916,
3.58957882764113));
#28146=CARTESIAN_POINT('Ctrl Pts',(-0.154316540000352,0.0159383321389732,
3.58876476376157));
#28147=CARTESIAN_POINT('Ctrl Pts',(-0.144808574808872,0.0829945710278969,
3.58530413985639));
#28148=CARTESIAN_POINT('Ctrl Pts',(-0.0479747871584019,0.175962994372803,
3.57919695592558));
#28149=CARTESIAN_POINT('Ctrl Pts',(0.121839171429706,0.13571993663382,3.5712572758487));
#28150=CARTESIAN_POINT('Ctrl Pts',(0.180099946935509,-0.0287862221383337,
3.56331759577183));
#28151=CARTESIAN_POINT('Ctrl Pts',(0.0734653204375665,-0.166934393666355,
3.55537791569495));
#28152=CARTESIAN_POINT('Ctrl Pts',(-0.0998464626320651,-0.152294592499083,
3.54746499298472));
#28153=CARTESIAN_POINT('Ctrl Pts',(-0.154507996889821,-0.0505553114913108,
3.54219863030011));
#28154=CARTESIAN_POINT('Ctrl Pts',(-0.154553716617854,1.07385516829459E-5,
3.53957882764113));
#28155=CARTESIAN_POINT('Origin',(0.,0.,4.11042117235887));
#28156=CARTESIAN_POINT('',(-0.154093198061062,-8.33060061860361E-5,3.63957882764113));
#28157=CARTESIAN_POINT('',(-0.154532949196129,5.22176212347235E-5,3.63542117235887));
#28158=CARTESIAN_POINT('',(-0.1543,7.47606542906876E-15,4.11042117235887));
#28159=CARTESIAN_POINT('Ctrl Pts',(-0.154532949196129,5.22176212347084E-5,
3.63542117235887));
#28160=CARTESIAN_POINT('Ctrl Pts',(-0.154545584588578,0.00292672178698735,
3.63527230200821));
#28161=CARTESIAN_POINT('Ctrl Pts',(-0.153169988902963,0.0568907246896308,
3.63247687163192));
#28162=CARTESIAN_POINT('Ctrl Pts',(-0.0901397813258339,0.158554191001936,
3.62703488123002));
#28163=CARTESIAN_POINT('Ctrl Pts',(0.0843490755327352,0.161709110561297,
3.61909520115314));
#28164=CARTESIAN_POINT('Ctrl Pts',(0.181609876119891,0.0168069020193158,
3.61115552107626));
#28165=CARTESIAN_POINT('Ctrl Pts',(0.11259272547993,-0.14348343554309,3.60321584099938));
#28166=CARTESIAN_POINT('Ctrl Pts',(-0.0595116136917225,-0.1724033835878,
3.59527616092251));
#28167=CARTESIAN_POINT('Ctrl Pts',(-0.147380741016298,-0.0760839947500021,
3.58934460470901));
#28168=CARTESIAN_POINT('Ctrl Pts',(-0.154401281957667,-0.0125195312047306,
3.58605960852113));
#28169=CARTESIAN_POINT('Ctrl Pts',(-0.154288256028425,-0.000141223516069763,
3.58542117235887));
#28170=CARTESIAN_POINT('Ctrl Pts',(-0.154093198061063,-8.33060061860274E-5,
3.63957882764113));
#28171=CARTESIAN_POINT('Ctrl Pts',(-0.153940587938977,0.0310641981069166,
3.63797745724865));
#28172=CARTESIAN_POINT('Ctrl Pts',(-0.129646233104354,0.113907608400038,
3.63372952683056));
#28173=CARTESIAN_POINT('Ctrl Pts',(0.00558664719359638,0.182300288895857,
3.62683503638684));
#28174=CARTESIAN_POINT('Ctrl Pts',(0.156205528517827,0.094151159125646,
3.61889535630996));
#28175=CARTESIAN_POINT('Ctrl Pts',(0.163806179027695,-0.0802006497663837,
3.61095567623308));
#28176=CARTESIAN_POINT('Ctrl Pts',(0.0214296163208854,-0.181122531330724,
3.60301599615621));
#28177=CARTESIAN_POINT('Ctrl Pts',(-0.123957687612568,-0.122868073634794,
3.59589037995889));
#28178=CARTESIAN_POINT('Ctrl Pts',(-0.1539078579151,-0.0354567255707862,
3.5914113237872));
#28179=CARTESIAN_POINT('Ctrl Pts',(-0.15419083216807,0.000129561635314916,
3.58957882764113));
#28180=CARTESIAN_POINT('Origin',(0.,0.,4.11042117235887));
#28181=CARTESIAN_POINT('',(-0.154494739391599,-8.56666717596894E-5,3.68957882764113));
#28182=CARTESIAN_POINT('',(-0.15413359010754,0.000108847378321225,3.68542117235887));
#28183=CARTESIAN_POINT('',(-0.1543,7.47606542906876E-15,4.11042117235887));
#28184=CARTESIAN_POINT('Ctrl Pts',(-0.15413359010754,0.00010884737832121,
3.68542117235887));
#28185=CARTESIAN_POINT('Ctrl Pts',(-0.154252061492927,0.0183060191525707,
3.6844849954953));
#28186=CARTESIAN_POINT('Ctrl Pts',(-0.142855501009428,0.0878027720491901,
3.6809022586061));
#28187=CARTESIAN_POINT('Ctrl Pts',(-0.039826269011209,0.177984489264188,
3.67467296169127));
#28188=CARTESIAN_POINT('Ctrl Pts',(0.127955809817362,0.129968921992697,
3.66673328161439));
#28189=CARTESIAN_POINT('Ctrl Pts',(0.178584458888466,-0.0370432344610292,
3.65879360153752));
#28190=CARTESIAN_POINT('Ctrl Pts',(0.0657052360091523,-0.170139449612234,
3.65085392146064));
#28191=CARTESIAN_POINT('Ctrl Pts',(-0.104087723049408,-0.147885095147454,
3.64306311173443));
#28192=CARTESIAN_POINT('Ctrl Pts',(-0.154320957425313,-0.0481751113503961,
3.63791886203384));
#28193=CARTESIAN_POINT('Ctrl Pts',(-0.154532949196129,5.22176212347084E-5,
3.63542117235887));
#28194=CARTESIAN_POINT('Ctrl Pts',(-0.154494739391599,-8.56666717596998E-5,
3.68957882764113));
#28195=CARTESIAN_POINT('Ctrl Pts',(-0.15418701910941,0.0460669561753479,
3.68719015073574));
#28196=CARTESIAN_POINT('Ctrl Pts',(-0.107714707332757,0.143892491682726,
3.68215491380472));
#28197=CARTESIAN_POINT('Ctrl Pts',(0.0586595287281965,0.172695299861449,
3.67447311684809));
#28198=CARTESIAN_POINT('Ctrl Pts',(0.176911729524118,0.0443491475303153,
3.66653343677121));
#28199=CARTESIAN_POINT('Ctrl Pts',(0.133187572742707,-0.124602076359984,
3.65859375669434));
#28200=CARTESIAN_POINT('Ctrl Pts',(-0.0324800977009374,-0.179470471240069,
3.65065407661746));
#28201=CARTESIAN_POINT('Ctrl Pts',(-0.140993802389242,-0.0920951181032393,
3.64431576693306));
#28202=CARTESIAN_POINT('Ctrl Pts',(-0.154192804322217,-0.0204127991394723,
3.64062401727428));
#28203=CARTESIAN_POINT('Ctrl Pts',(-0.154093198061063,-8.33060061860274E-5,
3.63957882764113));
#28204=CARTESIAN_POINT('Origin',(0.,0.,4.11042117235887));
#28205=CARTESIAN_POINT('',(-0.154352374546534,0.000136543067356262,3.73957882764113));
#28206=CARTESIAN_POINT('',(-0.154139174508622,-0.000111501026995055,3.73542117235887));
#28207=CARTESIAN_POINT('',(-0.1543,7.47606542906876E-15,4.11042117235887));
#28208=CARTESIAN_POINT('Ctrl Pts',(-0.154139174508622,-0.000111501026995059,
3.73542117235887));
#28209=CARTESIAN_POINT('Ctrl Pts',(-0.153915233552703,0.0333860868580806,
3.73369768898238));
#28210=CARTESIAN_POINT('Ctrl Pts',(-0.1267153517394,0.118653316414882,3.72932764558026));
#28211=CARTESIAN_POINT('Ctrl Pts',(0.0139700521550768,0.18185006934563,
3.72231104215253));
#28212=CARTESIAN_POINT('Ctrl Pts',(0.160372810275332,0.0868629483698537,
3.71437136207565));
#28213=CARTESIAN_POINT('Ctrl Pts',(0.15994186929589,-0.087653913339944,
3.70643168199877));
#28214=CARTESIAN_POINT('Ctrl Pts',(0.013071788942189,-0.181916844788939,
3.6984920019219));
#28215=CARTESIAN_POINT('Ctrl Pts',(-0.127037714877433,-0.11814535336758,
3.6914884987086));
#28216=CARTESIAN_POINT('Ctrl Pts',(-0.153917144400928,-0.0331371528280101,
3.68713155552092));
#28217=CARTESIAN_POINT('Ctrl Pts',(-0.15413359010754,0.00010884737832121,
3.68542117235887));
#28218=CARTESIAN_POINT('Ctrl Pts',(-0.154352374546534,0.000136543067356257,
3.73957882764113));
#28219=CARTESIAN_POINT('Ctrl Pts',(-0.154446737273245,0.0103903099163322,
3.73904940424845));
#28220=CARTESIAN_POINT('Ctrl Pts',(-0.148841316561083,0.0717994892151511,
3.73587342083015));
#28221=CARTESIAN_POINT('Ctrl Pts',(-0.0665446905722607,0.169812870767156,
3.73005087738622));
#28222=CARTESIAN_POINT('Ctrl Pts',(0.106602640202898,0.147988121222216,
3.72211119730934));
#28223=CARTESIAN_POINT('Ctrl Pts',(0.182147017152552,-0.0093311876933208,
3.71417151723247));
#28224=CARTESIAN_POINT('Ctrl Pts',(0.0909217261957518,-0.158107073301583,
3.70623183715559));
#28225=CARTESIAN_POINT('Ctrl Pts',(-0.0835494302172658,-0.162123717048593,
3.69829215707872));
#28226=CARTESIAN_POINT('Ctrl Pts',(-0.152048491522357,-0.0611528114853893,
3.69274115390723));
#28227=CARTESIAN_POINT('Ctrl Pts',(-0.154527961074428,-0.00506833400535766,
3.68983671076137));
#28228=CARTESIAN_POINT('Ctrl Pts',(-0.154494739391599,-8.56666717596998E-5,
3.68957882764113));
#28229=CARTESIAN_POINT('Origin',(0.,0.,4.11042117235887));
#28230=CARTESIAN_POINT('',(-0.154047977067031,2.09413777367551E-6,3.78957882764113));
#28231=CARTESIAN_POINT('',(-0.154536408180499,-4.7848165513455E-5,3.78542117235887));
#28232=CARTESIAN_POINT('',(-0.1543,7.47606542906876E-15,4.11042117235887));
#28233=CARTESIAN_POINT('Ctrl Pts',(-0.154536408180499,-4.78481655134459E-5,
3.78542117235887));
#28234=CARTESIAN_POINT('Ctrl Pts',(-0.154339106087067,0.0484295369338371,
3.78291038246947));
#28235=CARTESIAN_POINT('Ctrl Pts',(-0.103641790719782,0.148361335894058,
3.77775303255443));
#28236=CARTESIAN_POINT('Ctrl Pts',(0.0665446937287967,0.169812878822259,
3.76994912261378));
#28237=CARTESIAN_POINT('Ctrl Pts',(0.178765223990991,0.0361608181406009,
3.7620094425369));
#28238=CARTESIAN_POINT('Ctrl Pts',(0.127312379282745,-0.130599265535886,
3.75406976246003));
#28239=CARTESIAN_POINT('Ctrl Pts',(-0.0407047855299705,-0.177785630781348,
3.74613008238315));
#28240=CARTESIAN_POINT('Ctrl Pts',(-0.143071654254016,-0.0872869087240706,
3.73991388568277));
#28241=CARTESIAN_POINT('Ctrl Pts',(-0.154259114549828,-0.0180524000230757,
3.73634424900801));
#28242=CARTESIAN_POINT('Ctrl Pts',(-0.154139174508622,-0.000111501026995059,
3.73542117235887));
#28243=CARTESIAN_POINT('Ctrl Pts',(-0.154047977067031,2.09413777367898E-6,
3.78957882764113));
#28244=CARTESIAN_POINT('Ctrl Pts',(-0.154051078605937,0.0256319813134887,
3.78826209773554));
#28245=CARTESIAN_POINT('Ctrl Pts',(-0.135851564244815,0.102772493157479,
3.78429880780432));
#28246=CARTESIAN_POINT('Ctrl Pts',(-0.013970051492431,0.181850060719556,
3.77768895784748));
#28247=CARTESIAN_POINT('Ctrl Pts',(0.145223361235896,0.110339395832533,
3.7697492777706));
#28248=CARTESIAN_POINT('Ctrl Pts',(0.171453565975463,-0.0621955113766863,
3.76180959769372));
#28249=CARTESIAN_POINT('Ctrl Pts',(0.0407047835991549,-0.177785622348059,
3.75386991761685));
#28250=CARTESIAN_POINT('Ctrl Pts',(-0.11610887230377,-0.133745678862782,
3.74645966093265));
#28251=CARTESIAN_POINT('Ctrl Pts',(-0.153975022906486,-0.0408677376689339,
3.74169596427408));
#28252=CARTESIAN_POINT('Ctrl Pts',(-0.154352374546534,0.000136543067356257,
3.73957882764113));
#28253=CARTESIAN_POINT('Origin',(0.,0.,4.11042117235887));
#28254=CARTESIAN_POINT('',(-0.154344683817836,-0.000137602699895489,3.83957882764113));
#28255=CARTESIAN_POINT('',(-0.154280621254558,0.000141160201694546,3.83542117235887));
#28256=CARTESIAN_POINT('',(-0.1543,7.47606542906876E-15,4.11042117235887));
#28257=CARTESIAN_POINT('Ctrl Pts',(-0.154280621254558,0.000141160201694572,
3.83542117235887));
#28258=CARTESIAN_POINT('Ctrl Pts',(-0.154395390544122,0.0127750301081681,
3.83476963598218));
#28259=CARTESIAN_POINT('Ctrl Pts',(-0.147198204620896,0.0765990159781269,
3.83147153957986));
#28260=CARTESIAN_POINT('Ctrl Pts',(-0.0586595315107243,0.172695308053416,
3.82552688315191));
#28261=CARTESIAN_POINT('Ctrl Pts',(0.113300008356683,0.142925568707939,
3.81758720307504));
#28262=CARTESIAN_POINT('Ctrl Pts',(0.181524636378177,-0.0177035721096275,
3.80964752299816));
#28263=CARTESIAN_POINT('Ctrl Pts',(0.0835494341804624,-0.162123724738966,
3.80170784292129));
#28264=CARTESIAN_POINT('Ctrl Pts',(-0.0909217305086156,-0.158107080801413,
3.7937681628444));
#28265=CARTESIAN_POINT('Ctrl Pts',(-0.15329856504372,-0.056379054482583,
3.78833927265694));
#28266=CARTESIAN_POINT('Ctrl Pts',(-0.154547077226211,-0.00266924679639216,
3.78555694249509));
#28267=CARTESIAN_POINT('Ctrl Pts',(-0.154536408180499,-4.78481655134459E-5,
3.78542117235887));
#28268=CARTESIAN_POINT('Ctrl Pts',(-0.154344683817836,-0.000137602699895493,
3.83957882764113));
#28269=CARTESIAN_POINT('Ctrl Pts',(-0.153968758841032,0.0406181785207979,
3.83747479122262));
#28270=CARTESIAN_POINT('Ctrl Pts',(-0.11649114353226,0.133249851238064,
3.83272419477849));
#28271=CARTESIAN_POINT('Ctrl Pts',(0.039826267121788,0.177984480821945,
3.82532703830873));
#28272=CARTESIAN_POINT('Ctrl Pts',(0.171144313607041,0.063041501012073,
3.81738735823185));
#28273=CARTESIAN_POINT('Ctrl Pts',(0.145766517224248,-0.109620843643728,
3.80944767815498));
#28274=CARTESIAN_POINT('Ctrl Pts',(-0.0130717883220708,-0.181916836159762,
3.8015079980781));
#28275=CARTESIAN_POINT('Ctrl Pts',(-0.135584681571728,-0.103286631626578,
3.79488504790682));
#28276=CARTESIAN_POINT('Ctrl Pts',(-0.154044844670753,-0.0258827861209538,
3.79090865776116));
#28277=CARTESIAN_POINT('Ctrl Pts',(-0.154047977067031,2.09413777367898E-6,
3.78957882764113));
#28278=CARTESIAN_POINT('Origin',(0.,0.,4.11042117235887));
#28279=CARTESIAN_POINT('',(-0.154500132216325,8.19700297638587E-5,3.88957882764113));
#28280=CARTESIAN_POINT('',(-0.154055933642351,-3.65432311820964E-5,3.88542117235887));
#28281=CARTESIAN_POINT('',(-0.1543,7.47606542906876E-15,4.11042117235887));
#28282=CARTESIAN_POINT('Ctrl Pts',(-0.154055933642351,-3.6543231182122E-5,
3.88542117235887));
#28283=CARTESIAN_POINT('Ctrl Pts',(-0.15399662440304,0.0279666460980613,
3.88398232946926));
#28284=CARTESIAN_POINT('Ctrl Pts',(-0.133294661580101,0.10755966601202,
3.87989692655402));
#28285=CARTESIAN_POINT('Ctrl Pts',(-0.005586647457645,0.182300297549597,
3.87316496361317));
#28286=CARTESIAN_POINT('Ctrl Pts',(0.150147248343024,0.103539432915148,
3.86522528353629));
#28287=CARTESIAN_POINT('Ctrl Pts',(0.168409737102627,-0.0700197873807462,
3.85728560345941));
#28288=CARTESIAN_POINT('Ctrl Pts',(0.0324800992415292,-0.179470479754251,
3.84934592338254));
#28289=CARTESIAN_POINT('Ctrl Pts',(-0.1195927593937,-0.129104626018084,
3.84205777968236));
#28290=CARTESIAN_POINT('Ctrl Pts',(-0.153929194296616,-0.0385441229881096,
3.8374161960078));
#28291=CARTESIAN_POINT('Ctrl Pts',(-0.154280621254558,0.000141160201694572,
3.83542117235887));
#28292=CARTESIAN_POINT('Ctrl Pts',(-0.154500132216325,8.19700297638379E-5,
3.88957882764113));
#28293=CARTESIAN_POINT('Ctrl Pts',(-0.1545305647953,0.00481108885999716,
3.88933404473533));
#28294=CARTESIAN_POINT('Ctrl Pts',(-0.152188184006249,0.0606402533846132,
3.88644270180391));
#28295=CARTESIAN_POINT('Ctrl Pts',(-0.0843490715154628,0.161709102853824,
3.88090479884686));
#28296=CARTESIAN_POINT('Ctrl Pts',(0.0901397770410241,0.158554183500776,
3.87296511876998));
#28297=CARTESIAN_POINT('Ctrl Pts',(0.182098715355847,0.0102306290122647,
3.86502543869311));
#28298=CARTESIAN_POINT('Ctrl Pts',(0.107332199369115,-0.147459841777235,
3.85708575861623));
#28299=CARTESIAN_POINT('Ctrl Pts',(-0.0657052328909015,-0.17013944154474,
3.84914607853936));
#28300=CARTESIAN_POINT('Ctrl Pts',(-0.148671156397415,-0.0723140833987834,
3.84331043488099));
#28301=CARTESIAN_POINT('Ctrl Pts',(-0.154441615683002,-0.0106464385947012,
3.84012135124824));
#28302=CARTESIAN_POINT('Ctrl Pts',(-0.154344683817836,-0.000137602699895493,
3.83957882764113));
#28303=CARTESIAN_POINT('Origin',(0.,0.,4.11042117235887));
#28304=CARTESIAN_POINT('',(-0.154097159264761,8.62650376686758E-5,3.93957882764113));
#28305=CARTESIAN_POINT('',(-0.154414683966261,-0.000122711940234539,3.93542117235887));
#28306=CARTESIAN_POINT('',(-0.1543,7.47606542906876E-15,4.11042117235887));
#28307=CARTESIAN_POINT('Ctrl Pts',(-0.154414683966261,-0.00012271194023455,
3.93542117235887));
#28308=CARTESIAN_POINT('Ctrl Pts',(-0.15404065948349,0.0429479512135688,
3.93319502295635));
#28309=CARTESIAN_POINT('Ctrl Pts',(-0.11284743018063,0.1378508358131,3.9283223135282));
#28310=CARTESIAN_POINT('Ctrl Pts',(0.0479747894892283,0.175963002958517,
3.92080304407442));
#28311=CARTESIAN_POINT('Ctrl Pts',(0.173864125597012,0.0550988560374321,
3.91286336399754));
#28312=CARTESIAN_POINT('Ctrl Pts',(0.140567423109983,-0.116212816074597,
3.90492368392067));
#28313=CARTESIAN_POINT('Ctrl Pts',(-0.0214296173447312,-0.181122539961793,
3.89698400384379));
#28314=CARTESIAN_POINT('Ctrl Pts',(-0.138004452641611,-0.0984898965999405,
3.89048316665653));
#28315=CARTESIAN_POINT('Ctrl Pts',(-0.154105715856349,-0.0235414942304966,
3.88662888949489));
#28316=CARTESIAN_POINT('Ctrl Pts',(-0.154055933642351,-3.6543231182122E-5,
3.88542117235887));
#28317=CARTESIAN_POINT('Ctrl Pts',(-0.154097159264761,8.62650376686723E-5,
3.93957882764113));
#28318=CARTESIAN_POINT('Ctrl Pts',(-0.154199890802351,0.0201598980625174,
3.93854673822241));
#28319=CARTESIAN_POINT('Ctrl Pts',(-0.141224360537215,0.0915805799143205,
3.93486808877808));
#28320=CARTESIAN_POINT('Ctrl Pts',(-0.0333654229848094,0.179306981584077,
3.92854287930812));
#28321=CARTESIAN_POINT('Ctrl Pts',(0.132570265831228,0.125258780485074,
3.92060319923124));
#28322=CARTESIAN_POINT('Ctrl Pts',(0.17712875926901,-0.0434751369680033,
3.91266351915436));
#28323=CARTESIAN_POINT('Ctrl Pts',(0.059511610779771,-0.172403375181386,
3.90472383907749));
#28324=CARTESIAN_POINT('Ctrl Pts',(-0.107286687880009,-0.144375040164272,
3.89702894190641));
#28325=CARTESIAN_POINT('Ctrl Pts',(-0.154201531823291,-0.0463195111784584,
3.89198060476095));
#28326=CARTESIAN_POINT('Ctrl Pts',(-0.154500132216325,8.19700297638379E-5,
3.88957882764113));
#28327=CARTESIAN_POINT('Origin',(0.,0.,4.11042117235887));
#28328=CARTESIAN_POINT('',(-0.154145398954164,-0.00018319008806407,3.98957882764113));
#28329=CARTESIAN_POINT('',(-0.154443265232512,0.000108744696557919,3.98542117235887));
#28330=CARTESIAN_POINT('',(-0.1543,7.47606542906876E-15,4.11042117235887));
#28331=CARTESIAN_POINT('',(-0.0398513841857263,-0.149064942821851,4.));
#28332=CARTESIAN_POINT('Ctrl Pts',(-0.0398513841857263,-0.149064942821851,
4.));
#28333=CARTESIAN_POINT('Ctrl Pts',(-0.0894268873061843,-0.13581130730129,
3.99735343997437));
#28334=CARTESIAN_POINT('Ctrl Pts',(-0.144571567721208,-0.0835405737349159,
3.99387971585475));
#28335=CARTESIAN_POINT('Ctrl Pts',(-0.154267320225706,-0.0162511224334367,
3.99040599173513));
#28336=CARTESIAN_POINT('Ctrl Pts',(-0.154145398954164,-0.000183190088064077,
3.98957882764113));
#28337=CARTESIAN_POINT('',(0.0399397509085001,-0.149330346493117,4.));
#28338=CARTESIAN_POINT('Origin',(0.,0.,4.));
#28339=CARTESIAN_POINT('Ctrl Pts',(0.0399398308045223,-0.149330586455588,
4.));
#28340=CARTESIAN_POINT('Ctrl Pts',(-0.00819994193508078,-0.162114963086391,
3.9974200549221));
#28341=CARTESIAN_POINT('Ctrl Pts',(-0.111773735607764,-0.138502981643238,
3.99256044570839));
#28342=CARTESIAN_POINT('Ctrl Pts',(-0.154082201487749,-0.0439653055987776,
3.98770083649468));
#28343=CARTESIAN_POINT('Ctrl Pts',(-0.154443265232512,0.000108744696557906,
3.98542117235887));
#28344=CARTESIAN_POINT('Origin',(-1.70916393953233E-17,-6.81365885416763E-18,
3.5));
#28345=CARTESIAN_POINT('Ctrl Pts',(-0.0958116152722498,0.0825211298936362,
3.5));
#28346=CARTESIAN_POINT('Ctrl Pts',(-0.100695982673166,0.0779597798732974,
3.5));
#28347=CARTESIAN_POINT('Ctrl Pts',(-0.105169094336774,0.073000191113619,
3.5));
#28348=CARTESIAN_POINT('Ctrl Pts',(-0.109227190160158,0.0677117533966587,
3.5));
#28349=CARTESIAN_POINT('Ctrl Pts',(-0.111694873825402,0.0644959122887171,
3.5));
#28350=CARTESIAN_POINT('Ctrl Pts',(-0.114010184214277,0.0611562073506752,
3.5));
#28351=CARTESIAN_POINT('Ctrl Pts',(-0.116166807098829,0.0577125335531249,
3.5));
#28352=CARTESIAN_POINT('Ctrl Pts',(-0.121431726365849,0.0493055632589991,
3.5));
#28353=CARTESIAN_POINT('Ctrl Pts',(-0.12573464769667,0.0403151423737322,
3.5));
#28354=CARTESIAN_POINT('Ctrl Pts',(-0.129045466546674,0.0309386517006337,
3.5));
#28355=CARTESIAN_POINT('Ctrl Pts',(-0.130207164312345,0.0276486353154881,
3.5));
#28356=CARTESIAN_POINT('Ctrl Pts',(-0.131243087485824,0.0243197585947972,
3.5));
#28357=CARTESIAN_POINT('Ctrl Pts',(-0.132152263806834,0.0209620064696601,
3.5));
#28358=CARTESIAN_POINT('Ctrl Pts',(-0.134828933182204,0.0110765837240964,
3.5));
#28359=CARTESIAN_POINT('Ctrl Pts',(-0.136412178238084,0.000939292992310017,
3.5));
#28360=CARTESIAN_POINT('Ctrl Pts',(-0.136856372906323,-0.00925247465139327,
3.5));
#28361=CARTESIAN_POINT('Ctrl Pts',(-0.137021913483504,-0.0130506992112034,
3.5));
#28362=CARTESIAN_POINT('Ctrl Pts',(-0.137028726314264,-0.0168567537781713,
3.5));
#28363=CARTESIAN_POINT('Ctrl Pts',(-0.136872398016052,-0.0206609891299379,
3.5));
#28364=CARTESIAN_POINT('Ctrl Pts',(-0.136740582821431,-0.0238687002674301,
3.5));
#28365=CARTESIAN_POINT('Ctrl Pts',(-0.136493094718847,-0.0270653690856263,
3.5));
#28366=CARTESIAN_POINT('Ctrl Pts',(-0.13612917734588,-0.0302430275614766,
3.5));
#28367=CARTESIAN_POINT('Ctrl Pts',(-0.13576659429471,-0.0334090349888054,
3.5));
#28368=CARTESIAN_POINT('Ctrl Pts',(-0.135288410857674,-0.0365568188154616,
3.5));
#28369=CARTESIAN_POINT('Ctrl Pts',(-0.134693327673148,-0.0396806409761667,
3.5));
#28370=CARTESIAN_POINT('Ctrl Pts',(-0.133341599676801,-0.0467763848654778,
3.5));
#28371=CARTESIAN_POINT('Ctrl Pts',(-0.131387825400402,-0.0537485551880799,
3.5));
#28372=CARTESIAN_POINT('Ctrl Pts',(-0.128888271219693,-0.0605519919600177,
3.5));
#28373=CARTESIAN_POINT('Ctrl Pts',(-0.127520602506107,-0.0642745948504241,
3.5));
#28374=CARTESIAN_POINT('Ctrl Pts',(-0.125989250183059,-0.0679466858359917,
3.5));
#28375=CARTESIAN_POINT('Ctrl Pts',(-0.124301567034569,-0.0715605953668731,
3.5));
#28376=CARTESIAN_POINT('Ctrl Pts',(-0.123083413065749,-0.0741690815877246,
3.5));
#28377=CARTESIAN_POINT('Ctrl Pts',(-0.121784536276434,-0.0767452222753887,
3.5));
#28378=CARTESIAN_POINT('Ctrl Pts',(-0.120412533496435,-0.0792783080753084,
3.5));
#28379=CARTESIAN_POINT('Ctrl Pts',(-0.116240621079353,-0.0869807794232376,
3.5));
#28380=CARTESIAN_POINT('Ctrl Pts',(-0.111384900653015,-0.0943068033536031,
3.5));
#28381=CARTESIAN_POINT('Ctrl Pts',(-0.105936294580107,-0.101180758720708,
3.5));
#28382=CARTESIAN_POINT('Ctrl Pts',(-0.102498213514854,-0.105518237972245,
3.5));
#28383=CARTESIAN_POINT('Ctrl Pts',(-0.0988234872002696,-0.109675688132788,
3.5));
#28384=CARTESIAN_POINT('Ctrl Pts',(-0.0949300211352312,-0.113632240993693,
3.5));
#28385=CARTESIAN_POINT('Ctrl Pts',(-0.0916236146803262,-0.116992221972066,
3.5));
#28386=CARTESIAN_POINT('Ctrl Pts',(-0.0881545091528211,-0.120210812929281,
3.5));
#28387=CARTESIAN_POINT('Ctrl Pts',(-0.0845585132916744,-0.123253141705618,
3.5));
#28388=CARTESIAN_POINT('Ctrl Pts',(-0.0763242263006133,-0.13021961475866,
3.5));
#28389=CARTESIAN_POINT('Ctrl Pts',(-0.0674109291876633,-0.136284624413674,
3.5));
#28390=CARTESIAN_POINT('Ctrl Pts',(-0.0579550193346048,-0.141304740223277,
3.5));
#28391=CARTESIAN_POINT('Ctrl Pts',(-0.0532842084112166,-0.143784460538354,
3.5));
#28392=CARTESIAN_POINT('Ctrl Pts',(-0.0484803425336181,-0.146008805046434,
3.5));
#28393=CARTESIAN_POINT('Ctrl Pts',(-0.0435567265409999,-0.147956912059339,
3.5));
#28394=CARTESIAN_POINT('Ctrl Pts',(-0.042358096554505,-0.148431169086302,
3.5));
#28395=CARTESIAN_POINT('Ctrl Pts',(-0.0411523620931259,-0.148889040418797,
3.5));
#28396=CARTESIAN_POINT('Ctrl Pts',(-0.0399398165374117,-0.14933059314829,
3.5));
#28397=CARTESIAN_POINT('Ctrl Pts',(0.0398513841857336,-0.149064942821849,
3.5));
#28398=CARTESIAN_POINT('Ctrl Pts',(0.0462529496128914,-0.146725837162888,
3.5));
#28399=CARTESIAN_POINT('Ctrl Pts',(0.0524692076951892,-0.14393427563735,
3.5));
#28400=CARTESIAN_POINT('Ctrl Pts',(0.0584702623153416,-0.140728485236784,
3.5));
#28401=CARTESIAN_POINT('Ctrl Pts',(0.0631250229031883,-0.138241891170577,
3.5));
#28402=CARTESIAN_POINT('Ctrl Pts',(0.0676502468975603,-0.1355058910355,
3.5));
#28403=CARTESIAN_POINT('Ctrl Pts',(0.0720296458894365,-0.132535875720451,
3.5));
#28404=CARTESIAN_POINT('Ctrl Pts',(0.0754784967726087,-0.130196938354537,
3.5));
#28405=CARTESIAN_POINT('Ctrl Pts',(0.0788293975632557,-0.127717841671465,
3.5));
#28406=CARTESIAN_POINT('Ctrl Pts',(0.0820734025861846,-0.125108353169529,
3.5));
#28407=CARTESIAN_POINT('Ctrl Pts',(0.0878699486728443,-0.120445592089575,
3.5));
#28408=CARTESIAN_POINT('Ctrl Pts',(0.0933277488655726,-0.115365506062939,
3.5));
#28409=CARTESIAN_POINT('Ctrl Pts',(0.0983983261001443,-0.109911369421357,
3.5));
#28410=CARTESIAN_POINT('Ctrl Pts',(0.100785232866561,-0.107343907167555,
3.5));
#28411=CARTESIAN_POINT('Ctrl Pts',(0.103082837759472,-0.104696811464977,
3.5));
#28412=CARTESIAN_POINT('Ctrl Pts',(0.105281553373082,-0.101981102913922,
3.5));
#28413=CARTESIAN_POINT('Ctrl Pts',(0.111767020079616,-0.0939706820648148,
3.5));
#28414=CARTESIAN_POINT('Ctrl Pts',(0.117410242387804,-0.0853491014404185,
3.5));
#28415=CARTESIAN_POINT('Ctrl Pts',(0.122076804303227,-0.0762334533122014,
3.5));
#28416=CARTESIAN_POINT('Ctrl Pts',(0.124156859535273,-0.0721702796253988,
3.5));
#28417=CARTESIAN_POINT('Ctrl Pts',(0.126042226032514,-0.0680087185900064,
3.5));
#28418=CARTESIAN_POINT('Ctrl Pts',(0.127717516401833,-0.0637585923271345,
3.5));
#28419=CARTESIAN_POINT('Ctrl Pts',(0.128878955464437,-0.0608120806339354,
3.5));
#28420=CARTESIAN_POINT('Ctrl Pts',(0.129938690733468,-0.0578239271836136,
3.5));
#28421=CARTESIAN_POINT('Ctrl Pts',(0.130888204891735,-0.0548097446101512,
3.5));
#28422=CARTESIAN_POINT('Ctrl Pts',(0.132091470075251,-0.0509900428017762,
3.5));
#28423=CARTESIAN_POINT('Ctrl Pts',(0.133119907502104,-0.0471234083998808,
3.5));
#28424=CARTESIAN_POINT('Ctrl Pts',(0.13396498302397,-0.0432168875268929,
3.5));
#28425=CARTESIAN_POINT('Ctrl Pts',(0.135449870731708,-0.03635271423797,
3.5));
#28426=CARTESIAN_POINT('Ctrl Pts',(0.136369320260194,-0.0293652097985063,
3.5));
#28427=CARTESIAN_POINT('Ctrl Pts',(0.136739868479968,-0.022319296125407,
3.5));
#28428=CARTESIAN_POINT('Ctrl Pts',(0.136938614931574,-0.0185401649189451,
3.5));
#28429=CARTESIAN_POINT('Ctrl Pts',(0.13697923643291,-0.0147442545690828,
3.5));
#28430=CARTESIAN_POINT('Ctrl Pts',(0.136862895918197,-0.0109420689853019,
3.5));
#28431=CARTESIAN_POINT('Ctrl Pts',(0.136768618157157,-0.00786092786453014,
3.5));
#28432=CARTESIAN_POINT('Ctrl Pts',(0.136571008887471,-0.00477673741219634,
3.5));
#28433=CARTESIAN_POINT('Ctrl Pts',(0.136272480032331,-0.00170755776859209,
3.5));
#28434=CARTESIAN_POINT('Ctrl Pts',(0.135524862167375,0.00597871273026037,
3.5));
#28435=CARTESIAN_POINT('Ctrl Pts',(0.134145273604047,0.0135925891081728,
3.5));
#28436=CARTESIAN_POINT('Ctrl Pts',(0.132154756111308,0.0210469694652312,
3.5));
#28437=CARTESIAN_POINT('Ctrl Pts',(0.130956639638983,0.0255338508563019,
3.5));
#28438=CARTESIAN_POINT('Ctrl Pts',(0.129536820205507,0.0299628465144204,
3.5));
#28439=CARTESIAN_POINT('Ctrl Pts',(0.127896985354882,0.0343130630344241,
3.5));
#28440=CARTESIAN_POINT('Ctrl Pts',(0.126764260724531,0.0373179981946284,
3.5));
#28441=CARTESIAN_POINT('Ctrl Pts',(0.125525608395292,0.0402872565072415,
3.5));
#28442=CARTESIAN_POINT('Ctrl Pts',(0.124183958141022,0.0432071171955597,
3.5));
#28443=CARTESIAN_POINT('Ctrl Pts',(0.120305951421964,0.0516469019546402,
3.5));
#28444=CARTESIAN_POINT('Ctrl Pts',(0.115595095267004,0.0596252551381628,
3.5));
#28445=CARTESIAN_POINT('Ctrl Pts',(0.110076005567125,0.0669787038662309,
3.5));
#28446=CARTESIAN_POINT('Ctrl Pts',(0.106491490638639,0.0717545905024268,
3.5));
#28447=CARTESIAN_POINT('Ctrl Pts',(0.102565240148127,0.0762663779558996,
3.5));
#28448=CARTESIAN_POINT('Ctrl Pts',(0.0982968917172504,0.0804596491219306,
3.5));
#28449=CARTESIAN_POINT('Ctrl Pts',(0.0975400014439711,0.081203226224454,
3.5));
#28450=CARTESIAN_POINT('Ctrl Pts',(0.0967723418961243,0.0819367632413509,
3.5));
#28451=CARTESIAN_POINT('Ctrl Pts',(0.0959941578858439,0.0826601402795114,
3.5));
#28452=CARTESIAN_POINT('Origin',(0.,0.,4.11042117235887));
#28453=CARTESIAN_POINT('Ctrl Pts',(-0.154443265232512,0.000108744696557909,
3.98542117235887));
#28454=CARTESIAN_POINT('Ctrl Pts',(-0.154501375899708,0.00720215273278324,
3.98505427646906));
#28455=CARTESIAN_POINT('Ctrl Pts',(-0.150833043785448,0.0654047280234095,
3.98204082055362));
#28456=CARTESIAN_POINT('Ctrl Pts',(-0.0768181153328184,0.165435267997838,
3.97638080461255));
#28457=CARTESIAN_POINT('Ctrl Pts',(0.0973408978391562,0.154229954870798,
3.96844112453568));
#28458=CARTESIAN_POINT('Ctrl Pts',(0.182376570303567,0.00184388772387479,
3.9605014444588));
#28459=CARTESIAN_POINT('Ctrl Pts',(0.100432518024861,-0.152245093163996,
3.95256176438192));
#28460=CARTESIAN_POINT('Ctrl Pts',(-0.0734653243360244,-0.166934402953208,
3.94462208430505));
#28461=CARTESIAN_POINT('Ctrl Pts',(-0.150201443282177,-0.0675205906017345,
3.9389085536307));
#28462=CARTESIAN_POINT('Ctrl Pts',(-0.154485318877682,-0.00825665133948968,
3.93584158298197));
#28463=CARTESIAN_POINT('Ctrl Pts',(-0.154414683966261,-0.00012271194023455,
3.93542117235887));
#28464=CARTESIAN_POINT('Ctrl Pts',(-0.154145398954164,-0.000183190088064077,
3.98957882764113));
#28465=CARTESIAN_POINT('Ctrl Pts',(-0.153877225967651,0.0351591693674689,
3.9877594317095));
#28466=CARTESIAN_POINT('Ctrl Pts',(-0.124353035696744,0.122445639808398,
3.98329347575225));
#28467=CARTESIAN_POINT('Ctrl Pts',(0.0205691872966891,0.181176549232701,
3.97618095976937));
#28468=CARTESIAN_POINT('Ctrl Pts',(0.16339053139201,0.0810339956098913,
3.9682412796925));
#28469=CARTESIAN_POINT('Ctrl Pts',(0.156677599794682,-0.0933915431448235,
3.96030159961562));
#28470=CARTESIAN_POINT('Ctrl Pts',(0.00648228676056323,-0.182263829019595,
3.95236191953875));
#28471=CARTESIAN_POINT('Ctrl Pts',(-0.129338242603737,-0.114419911622588,
3.94545432888058));
#28472=CARTESIAN_POINT('Ctrl Pts',(-0.153936458995158,-0.0313143964796836,
3.94119329824804));
#28473=CARTESIAN_POINT('Ctrl Pts',(-0.154097159264761,8.62650376686723E-5,
3.93957882764113));
#28474=CARTESIAN_POINT('Ctrl Pts',(0.095811615272233,0.0825211298936557,
4.));
#28475=CARTESIAN_POINT('Ctrl Pts',(0.123256207240687,0.0506564342651108,
3.99735343997437));
#28476=CARTESIAN_POINT('Ctrl Pts',(0.143368215702842,-0.042067892211591,
3.99206031992312));
#28477=CARTESIAN_POINT('Ctrl Pts',(0.0422170408642446,-0.143478264550263,
3.98412063984626));
#28478=CARTESIAN_POINT('Ctrl Pts',(-0.0975844110283061,-0.113165467831369,
3.97618095976937));
#28479=CARTESIAN_POINT('Ctrl Pts',(-0.148038914743343,0.0205825766583269,
3.9682412796925));
#28480=CARTESIAN_POINT('Ctrl Pts',(-0.0629530180417037,0.135575435115532,
3.96030159961561));
#28481=CARTESIAN_POINT('Ctrl Pts',(0.0797715912622248,0.126392597494572,
3.95236191953875));
#28482=CARTESIAN_POINT('Ctrl Pts',(0.149458958618833,0.00151107973223563,
3.94442223946186));
#28483=CARTESIAN_POINT('Ctrl Pts',(0.0823051970462972,-0.124765988532646,
3.936482559385));
#28484=CARTESIAN_POINT('Ctrl Pts',(-0.0602053808314341,-0.136803987384531,
3.92854287930812));
#28485=CARTESIAN_POINT('Ctrl Pts',(-0.147593255628917,-0.0235905240738923,
3.92060319923124));
#28486=CARTESIAN_POINT('Ctrl Pts',(-0.0998481138804565,0.11122350451698,
3.91266351915437));
#28487=CARTESIAN_POINT('Ctrl Pts',(0.0393156975431816,0.144202992379161,
3.90472383907749));
#28488=CARTESIAN_POINT('Ctrl Pts',(0.142482946738445,0.0451539231751995,
3.89678415900061));
#28489=CARTESIAN_POINT('Ctrl Pts',(0.115196050889548,-0.0952372689088321,
3.88884447892374));
#28490=CARTESIAN_POINT('Ctrl Pts',(-0.0175617311292369,-0.148431271407445,
3.88090479884687));
#28491=CARTESIAN_POINT('Ctrl Pts',(-0.134240390927499,-0.0657250333201687,
3.87296511876998));
#28492=CARTESIAN_POINT('Ctrl Pts',(-0.128011600896121,0.0771575802637476,
3.86502543869311));
#28493=CARTESIAN_POINT('Ctrl Pts',(-0.00457829922889965,0.149396452528493,
3.85708575861623));
#28494=CARTESIAN_POINT('Ctrl Pts',(0.123046789066594,0.0848513369547663,
3.84914607853936));
#28495=CARTESIAN_POINT('Ctrl Pts',(0.138013034715666,-0.0573817376169498,
3.84120639846248));
#28496=CARTESIAN_POINT('Ctrl Pts',(0.0266176834030549,-0.147077395754537,
3.83326671838561));
#28497=CARTESIAN_POINT('Ctrl Pts',(-0.109148213688832,-0.102112335081275,
3.82532703830873));
#28498=CARTESIAN_POINT('Ctrl Pts',(-0.144980487747744,0.0363444586596486,
3.81738735823185));
#28499=CARTESIAN_POINT('Ctrl Pts',(-0.0480719232633252,0.141525092050256,
3.80944767815498));
#28500=CARTESIAN_POINT('Ctrl Pts',(0.0928502012748058,0.117128568782365,
3.8015079980781));
#28501=CARTESIAN_POINT('Ctrl Pts',(0.148760792417501,-0.0145082092888036,
3.79356831800123));
#28502=CARTESIAN_POINT('Ctrl Pts',(0.0684693840059589,-0.13286160073391,
3.78562863792435));
#28503=CARTESIAN_POINT('Ctrl Pts',(-0.0745110357927053,-0.129569931090983,
3.77768895784747));
#28504=CARTESIAN_POINT('Ctrl Pts',(-0.149270845181396,-0.00764697822290441,
3.7697492777706));
#28505=CARTESIAN_POINT('Ctrl Pts',(-0.0873616623012301,0.121277374051889,
3.76180959769372));
#28506=CARTESIAN_POINT('Ctrl Pts',(0.0545338724692569,0.139162919812538,
3.75386991761685));
#28507=CARTESIAN_POINT('Ctrl Pts',(0.146499433400264,0.0296340599732921,
3.74593023753997));
#28508=CARTESIAN_POINT('Ctrl Pts',(0.104333443683106,-0.107027071464762,
3.7379905574631));
#28509=CARTESIAN_POINT('Ctrl Pts',(-0.0333578751151315,-0.14569664946404,
3.73005087738622));
#28510=CARTESIAN_POINT('Ctrl Pts',(-0.14050748182764,-0.0509696875349592,
3.72211119730934));
#28511=CARTESIAN_POINT('Ctrl Pts',(-0.119011632529845,0.0904239615350441,
3.71417151723247));
#28512=CARTESIAN_POINT('Ctrl Pts',(0.0114485618600744,0.149027487159785,
3.70623183715559));
#28513=CARTESIAN_POINT('Ctrl Pts',(0.131426713281372,0.0711848335798314,
3.69829215707872));
#28514=CARTESIAN_POINT('Ctrl Pts',(0.131073553936911,-0.0718330352678932,
3.69035247700184));
#28515=CARTESIAN_POINT('Ctrl Pts',(0.0107124284623447,-0.149082210133256,
3.68241279692496));
#28516=CARTESIAN_POINT('Ctrl Pts',(-0.119456752931603,-0.0898351026331364,
3.67447311684809));
#28517=CARTESIAN_POINT('Ctrl Pts',(-0.140254047194737,0.0516629823793918,
3.66653343677121));
#28518=CARTESIAN_POINT('Ctrl Pts',(-0.0326379242804108,0.145859615472823,
3.65859375669434));
#28519=CARTESIAN_POINT('Ctrl Pts',(0.10486073980172,0.10651050023316,3.65065407661746));
#28520=CARTESIAN_POINT('Ctrl Pts',(0.146351295051501,-0.0303572067245441,
3.64271439654059));
#28521=CARTESIAN_POINT('Ctrl Pts',(0.0538459306115186,-0.139430547008859,
3.63477471646371));
#28522=CARTESIAN_POINT('Ctrl Pts',(-0.0879595415059408,-0.12084444509365,
3.62683503638684));
#28523=CARTESIAN_POINT('Ctrl Pts',(-0.149231261493045,0.00838407713103302,
3.61889535630996));
#28524=CARTESIAN_POINT('Ctrl Pts',(-0.0738702226095378,0.12993634123263,
3.61095567623308));
#28525=CARTESIAN_POINT('Ctrl Pts',(0.0691246960538845,0.132521821325185,
3.60301599615621));
#28526=CARTESIAN_POINT('Ctrl Pts',(0.148830647021129,0.0137733814668988,
3.59507631607933));
#28527=CARTESIAN_POINT('Ctrl Pts',(0.0922705776859184,-0.11758574481156,
3.58713663600245));
#28528=CARTESIAN_POINT('Ctrl Pts',(-0.0487702109612334,-0.141285857774966,
3.57919695592558));
#28529=CARTESIAN_POINT('Ctrl Pts',(-0.145158345123895,-0.0356282001147357,
3.5712572758487));
#28530=CARTESIAN_POINT('Ctrl Pts',(-0.108642326262961,0.10265050841275,
3.56331759577183));
#28531=CARTESIAN_POINT('Ctrl Pts',(0.0273432144577738,0.14694341587319,
3.55537791569495));
#28532=CARTESIAN_POINT('Ctrl Pts',(0.138295730077318,0.0567008676982971,
3.54743823561807));
#28533=CARTESIAN_POINT('Ctrl Pts',(0.122624304118183,-0.0854607729482632,
3.5394985555412));
#28534=CARTESIAN_POINT('Ctrl Pts',(-0.00531228376040394,-0.149366579646122,
3.53155887546432));
#28535=CARTESIAN_POINT('Ctrl Pts',(-0.128398465432132,-0.0765350583850204,
3.52361919538745));
#28536=CARTESIAN_POINT('Ctrl Pts',(-0.133899765542225,0.0664079477775043,
3.51567951531057));
#28537=CARTESIAN_POINT('Ctrl Pts',(-0.0168566046022346,0.148475571278638,
3.5077398352337));
#28538=CARTESIAN_POINT('Ctrl Pts',(0.115720245650148,0.0947476421044766,
3.49980015515682));
#28539=CARTESIAN_POINT('Ctrl Pts',(0.142146925240749,-0.0460261281615502,
3.49186047507995));
#28540=CARTESIAN_POINT('Ctrl Pts',(0.0732860006472317,-0.111298378536925,
3.48656735502869));
#28541=CARTESIAN_POINT('Ctrl Pts',(0.0326585063531174,-0.122159831625553,
3.48392079500307));
#28542=CARTESIAN_POINT('Ctrl Pts',(0.102845629995659,0.0885794229410745,
4.00535973499898));
#28543=CARTESIAN_POINT('Ctrl Pts',(0.132305068112318,0.0543753790239966,
4.00271317497335));
#28544=CARTESIAN_POINT('Ctrl Pts',(0.153893600722808,-0.0451563087084747,
3.9974200549221));
#28545=CARTESIAN_POINT('Ctrl Pts',(0.0453164071172279,-0.154011728812092,
3.98948037484522));
#28546=CARTESIAN_POINT('Ctrl Pts',(-0.104748575644461,-0.121473516543913,
3.98154069476835));
#28547=CARTESIAN_POINT('Ctrl Pts',(-0.158907199376537,0.0220936475952833,
3.97360101469147));
#28548=CARTESIAN_POINT('Ctrl Pts',(-0.067574717138742,0.145528712742967,
3.9656613346146));
#28549=CARTESIAN_POINT('Ctrl Pts',(0.0856280267878686,0.135671716619981,
3.95772165453772));
#28550=CARTESIAN_POINT('Ctrl Pts',(0.160431495847078,0.00162201572944855,
3.94978197446085));
#28551=CARTESIAN_POINT('Ctrl Pts',(0.0883476373724852,-0.133925690076429,
3.94184229438397));
#28552=CARTESIAN_POINT('Ctrl Pts',(-0.0646253619996309,-0.146847459240757,
3.93390261430709));
#28553=CARTESIAN_POINT('Ctrl Pts',(-0.158428822175023,-0.0253224236269645,
3.92596293423022));
#28554=CARTESIAN_POINT('Ctrl Pts',(-0.107178468359357,0.119388983891694,
3.91802325415334));
#28555=CARTESIAN_POINT('Ctrl Pts',(0.0422020615251973,0.15478966257228,
3.91008357407647));
#28556=CARTESIAN_POINT('Ctrl Pts',(0.152943339691301,0.0484689007959436,
3.90214389399959));
#28557=CARTESIAN_POINT('Ctrl Pts',(0.123653174963026,-0.102229117964087,
3.89420421392272));
#28558=CARTESIAN_POINT('Ctrl Pts',(-0.0188510265344017,-0.159328360925561,
3.88626453384584));
#28559=CARTESIAN_POINT('Ctrl Pts',(-0.144095656216364,-0.0705502400631941,
3.87832485376896));
#28560=CARTESIAN_POINT('Ctrl Pts',(-0.137409579240545,0.0828221080358456,
3.87038517369209));
#28561=CARTESIAN_POINT('Ctrl Pts',(-0.00491441530514796,0.160364400868861,
3.86244549361521));
#28562=CARTESIAN_POINT('Ctrl Pts',(0.13208027549207,0.0910807022748934,
3.85450581353834));
#28563=CARTESIAN_POINT('Ctrl Pts',(0.148145268844653,-0.0615944208715485,
3.84656613346146));
#28564=CARTESIAN_POINT('Ctrl Pts',(0.0285718220158795,-0.157875090421108,
3.83862645338458));
#28565=CARTESIAN_POINT('Ctrl Pts',(-0.117161335479353,-0.109608917477515,
3.83068677330771));
#28566=CARTESIAN_POINT('Ctrl Pts',(-0.155624237803826,0.0390126889843388,
3.82274709323083));
#28567=CARTESIAN_POINT('Ctrl Pts',(-0.0516011260124583,0.151915164051309,
3.81480741315396));
#28568=CARTESIAN_POINT('Ctrl Pts',(0.0996668036354316,0.125727568757556,
3.80686773307708));
#28569=CARTESIAN_POINT('Ctrl Pts',(0.159682073737726,-0.0155733302290782,
3.7989280530002));
#28570=CARTESIAN_POINT('Ctrl Pts',(0.0734960673974602,-0.142615642068929,
3.79098837292333));
#28571=CARTESIAN_POINT('Ctrl Pts',(-0.0799812673646754,-0.139082314327793,
3.78304869284645));
#28572=CARTESIAN_POINT('Ctrl Pts',(-0.160229572051837,-0.00820838152726148,
3.77510901276958));
#28573=CARTESIAN_POINT('Ctrl Pts',(-0.0937753232873622,0.13018095878194,
3.7671693326927));
#28574=CARTESIAN_POINT('Ctrl Pts',(0.0585374795557702,0.149379572815778,
3.75922965261583));
#28575=CARTESIAN_POINT('Ctrl Pts',(0.157254696930506,0.0318096460290618,
3.75128997253895));
#28576=CARTESIAN_POINT('Ctrl Pts',(0.111993088882986,-0.11488446948847,
3.74335029246207));
#28577=CARTESIAN_POINT('Ctrl Pts',(-0.0358068452534112,-0.156392976569809,
3.7354106123852));
#28578=CARTESIAN_POINT('Ctrl Pts',(-0.15082284592122,-0.0547116297989597,
3.72747093230832));
#28579=CARTESIAN_POINT('Ctrl Pts',(-0.127748877728095,0.0970624413788584,
3.71953125223145));
#28580=CARTESIAN_POINT('Ctrl Pts',(0.0122890586250752,0.1599683478884,3.71159157215457));
#28581=CARTESIAN_POINT('Ctrl Pts',(0.141075412279359,0.0764108718431722,
3.7036518920777));
#28582=CARTESIAN_POINT('Ctrl Pts',(0.140696325723237,-0.0771066612919101,
3.69571221200082));
#28583=CARTESIAN_POINT('Ctrl Pts',(0.0114988819556263,-0.160027088351817,
3.68777253192394));
#28584=CARTESIAN_POINT('Ctrl Pts',(-0.128226676667323,-0.0964303513700096,
3.67983285184707));
#28585=CARTESIAN_POINT('Ctrl Pts',(-0.150550805371548,0.0554558229204912,
3.67189317177019));
#28586=CARTESIAN_POINT('Ctrl Pts',(-0.035034039190677,0.156567906736611,
3.66395349169332));
#28587=CARTESIAN_POINT('Ctrl Pts',(0.112559096473601,0.114329974153006,
3.65601381161644));
#28588=CARTESIAN_POINT('Ctrl Pts',(0.157095682997156,-0.0325858826367059,
3.64807413153956));
#28589=CARTESIAN_POINT('Ctrl Pts',(0.0577990324107298,-0.14966684787665,
3.64013445146269));
#28590=CARTESIAN_POINT('Ctrl Pts',(-0.0944170958250141,-0.129716246321693,
3.63219477138581));
#28591=CARTESIAN_POINT('Ctrl Pts',(-0.160187082324945,0.00899959459010582,
3.62425509130894));
#28592=CARTESIAN_POINT('Ctrl Pts',(-0.0792934088483033,0.139475624489065,
3.61631541123206));
#28593=CARTESIAN_POINT('Ctrl Pts',(0.0741994892135014,0.142250917737222,
3.60837573115519));
#28594=CARTESIAN_POINT('Ctrl Pts',(0.159757056720716,0.0147845549843712,
3.60043605107831));
#28595=CARTESIAN_POINT('Ctrl Pts',(0.099044626950589,-0.126218308388737,
3.59249637100143));
#28596=CARTESIAN_POINT('Ctrl Pts',(-0.0523506785380631,-0.151658366379244,
3.58455669092456));
#28597=CARTESIAN_POINT('Ctrl Pts',(-0.155815152588506,-0.0382438462810607,
3.57661701084768));
#28598=CARTESIAN_POINT('Ctrl Pts',(-0.116618308301774,0.110186600832138,
3.5686773307708));
#28599=CARTESIAN_POINT('Ctrl Pts',(0.0293506179707539,0.157731274399797,
3.56073765069393));
#28600=CARTESIAN_POINT('Ctrl Pts',(0.148448718300998,0.06086356485237,3.55279797061705));
#28601=CARTESIAN_POINT('Ctrl Pts',(0.131626773789177,-0.0917348800435817,
3.54485829054018));
#28602=CARTESIAN_POINT('Ctrl Pts',(-0.00570228534924597,-0.160332334867275,
3.5369186104633));
#28603=CARTESIAN_POINT('Ctrl Pts',(-0.137824845456608,-0.0821538836809814,
3.52897893038643));
#28604=CARTESIAN_POINT('Ctrl Pts',(-0.143730023800696,0.0712832907209694,
3.52103925030955));
#28605=CARTESIAN_POINT('Ctrl Pts',(-0.0180941331067087,0.159375913074104,
3.51309957023267));
#28606=CARTESIAN_POINT('Ctrl Pts',(0.124215853509266,0.101703545182399,
3.5051598901558));
#28607=CARTESIAN_POINT('Ctrl Pts',(0.152582649157857,-0.0494051387567767,
3.49722021007893));
#28608=CARTESIAN_POINT('Ctrl Pts',(0.0786662962002181,-0.119469354791712,
3.49192709002767));
#28609=CARTESIAN_POINT('Ctrl Pts',(0.0350561322973228,-0.131128202024318,
3.48928053000205));
#28610=CARTESIAN_POINT('Ctrl Pts',(0.109879644719085,0.0946377159884933,
4.01071946999795));
#28611=CARTESIAN_POINT('Ctrl Pts',(0.141353928983949,0.0580943237828825,
4.00807290997233));
#28612=CARTESIAN_POINT('Ctrl Pts',(0.164418985742774,-0.0482447252053583,
4.00277978992107));
#28613=CARTESIAN_POINT('Ctrl Pts',(0.0484157733702112,-0.164545193073921,
3.99484010984421));
#28614=CARTESIAN_POINT('Ctrl Pts',(-0.111912740260616,-0.129781565256457,
3.98690042976732));
#28615=CARTESIAN_POINT('Ctrl Pts',(-0.16977548400973,0.0236047185322397,
3.97896074969046));
#28616=CARTESIAN_POINT('Ctrl Pts',(-0.0721964162357802,0.155481990370402,
3.97102106961357));
#28617=CARTESIAN_POINT('Ctrl Pts',(0.0914844623135124,0.14495083574539,
3.9630813895367));
#28618=CARTESIAN_POINT('Ctrl Pts',(0.171404033075322,0.0017329517266617,
3.95514170945982));
#28619=CARTESIAN_POINT('Ctrl Pts',(0.0943900776986731,-0.143085391620212,
3.94720202938295));
#28620=CARTESIAN_POINT('Ctrl Pts',(-0.0690453431678277,-0.156890931096983,
3.93926234930607));
#28621=CARTESIAN_POINT('Ctrl Pts',(-0.169264388721129,-0.0270543231800365,
3.9313226692292));
#28622=CARTESIAN_POINT('Ctrl Pts',(-0.114508822838256,0.127554463266409,
3.92338298915232));
#28623=CARTESIAN_POINT('Ctrl Pts',(0.0450884255072127,0.165376332765398,
3.91544330907545));
#28624=CARTESIAN_POINT('Ctrl Pts',(0.163403732644156,0.0517838784166879,
3.90750362899857));
#28625=CARTESIAN_POINT('Ctrl Pts',(0.132110299036504,-0.109220967019342,
3.89956394892169));
#28626=CARTESIAN_POINT('Ctrl Pts',(-0.0201403219395664,-0.170225450443677,
3.89162426884482));
#28627=CARTESIAN_POINT('Ctrl Pts',(-0.153950921505229,-0.0753754468062197,
3.88368458876794));
#28628=CARTESIAN_POINT('Ctrl Pts',(-0.146807557584968,0.0884866358079437,
3.87574490869107));
#28629=CARTESIAN_POINT('Ctrl Pts',(-0.00525053138139654,0.171332349209229,
3.86780522861419));
#28630=CARTESIAN_POINT('Ctrl Pts',(0.141113761917547,0.0973100675950205,
3.85986554853731));
#28631=CARTESIAN_POINT('Ctrl Pts',(0.15827750297364,-0.0658071041261473,
3.85192586846044));
#28632=CARTESIAN_POINT('Ctrl Pts',(0.0305259606287044,-0.16867278508768,
3.84398618838356));
#28633=CARTESIAN_POINT('Ctrl Pts',(-0.125174457269873,-0.117105499873754,
3.83604650830669));
#28634=CARTESIAN_POINT('Ctrl Pts',(-0.166267987859908,0.0416809193090289,
3.82810682822981));
#28635=CARTESIAN_POINT('Ctrl Pts',(-0.0551303287615912,0.162305236052362,
3.82016714815293));
#28636=CARTESIAN_POINT('Ctrl Pts',(0.106483405996057,0.134326568732747,
3.81222746807606));
#28637=CARTESIAN_POINT('Ctrl Pts',(0.170603355057952,-0.0166384511693528,
3.80428778799918));
#28638=CARTESIAN_POINT('Ctrl Pts',(0.0785227507889612,-0.152369683403947,
3.79634810792231));
#28639=CARTESIAN_POINT('Ctrl Pts',(-0.0854514989366454,-0.148594697564603,
3.78840842784543));
#28640=CARTESIAN_POINT('Ctrl Pts',(-0.171188298922279,-0.00876978483161878,
3.78046874776855));
#28641=CARTESIAN_POINT('Ctrl Pts',(-0.100188984273494,0.139084543511992,
3.77252906769168));
#28642=CARTESIAN_POINT('Ctrl Pts',(0.0625410866422834,0.159596225819019,
3.7645893876148));
#28643=CARTESIAN_POINT('Ctrl Pts',(0.168009960460748,0.0339852320848313,
3.75664970753793));
#28644=CARTESIAN_POINT('Ctrl Pts',(0.119652734082865,-0.122741867512178,
3.74871002746105));
#28645=CARTESIAN_POINT('Ctrl Pts',(-0.0382558153916907,-0.167089303675579,
3.74077034738417));
#28646=CARTESIAN_POINT('Ctrl Pts',(-0.161138210014801,-0.0584535720629604,
3.7328306673073));
#28647=CARTESIAN_POINT('Ctrl Pts',(-0.136486122926345,0.103700921222673,
3.72489098723042));
#28648=CARTESIAN_POINT('Ctrl Pts',(0.0131295553900761,0.170909208617015,
3.71695130715355));
#28649=CARTESIAN_POINT('Ctrl Pts',(0.150724111277345,0.081636910106513,
3.70901162707667));
#28650=CARTESIAN_POINT('Ctrl Pts',(0.150319097509564,-0.0823802873159272,
3.7010719469998));
#28651=CARTESIAN_POINT('Ctrl Pts',(0.0122853354489075,-0.170971966570378,
3.69313226692292));
#28652=CARTESIAN_POINT('Ctrl Pts',(-0.136996600403042,-0.103025600106883,
3.68519258684605));
#28653=CARTESIAN_POINT('Ctrl Pts',(-0.16084756354836,0.0592486634615907,
3.67725290676916));
#28654=CARTESIAN_POINT('Ctrl Pts',(-0.037430154100943,0.1672761980004,3.66931322669229));
#28655=CARTESIAN_POINT('Ctrl Pts',(0.120257453145481,0.122149448072851,
3.66137354661541));
#28656=CARTESIAN_POINT('Ctrl Pts',(0.167840070942811,-0.0348145585488677,
3.65343386653854));
#28657=CARTESIAN_POINT('Ctrl Pts',(0.0617521342099411,-0.159903148744442,
3.64549418646166));
#28658=CARTESIAN_POINT('Ctrl Pts',(-0.100874650144087,-0.138588047549736,
3.63755450638479));
#28659=CARTESIAN_POINT('Ctrl Pts',(-0.171142903156845,0.00961511204917869,
3.62961482630791));
#28660=CARTESIAN_POINT('Ctrl Pts',(-0.0847165950870686,0.149014907745501,
3.62167514623104));
#28661=CARTESIAN_POINT('Ctrl Pts',(0.0792742823731183,0.15198001414926,
3.61373546615416));
#28662=CARTESIAN_POINT('Ctrl Pts',(0.170683466420304,0.0157957285018435,
3.60579578607728));
#28663=CARTESIAN_POINT('Ctrl Pts',(0.10581867621526,-0.134850871965913,
3.59785610600041));
#28664=CARTESIAN_POINT('Ctrl Pts',(-0.0559311461148929,-0.162030874983522,
3.58991642592353));
#28665=CARTESIAN_POINT('Ctrl Pts',(-0.166471960053118,-0.0408594924473857,
3.58197674584666));
#28666=CARTESIAN_POINT('Ctrl Pts',(-0.124594290340586,0.117722693251527,
3.57403706576978));
#28667=CARTESIAN_POINT('Ctrl Pts',(0.0313580214837342,0.168519132926404,
3.56609738569291));
#28668=CARTESIAN_POINT('Ctrl Pts',(0.158601706524679,0.065026262006443,
3.55815770561603));
#28669=CARTESIAN_POINT('Ctrl Pts',(0.14062924346017,-0.0980089871389004,
3.55021802553916));
#28670=CARTESIAN_POINT('Ctrl Pts',(-0.00609228693808808,-0.171298090088428,
3.54227834546228));
#28671=CARTESIAN_POINT('Ctrl Pts',(-0.147251225481083,-0.0877727089769424,
3.5343386653854));
#28672=CARTESIAN_POINT('Ctrl Pts',(-0.153560282059167,0.0761586336644345,
3.52639898530853));
#28673=CARTESIAN_POINT('Ctrl Pts',(-0.0193316616111828,0.17027625486957,
3.51845930523165));
#28674=CARTESIAN_POINT('Ctrl Pts',(0.132711461368385,0.10865944826032,3.51051962515478));
#28675=CARTESIAN_POINT('Ctrl Pts',(0.163018373074965,-0.0527841493520032,
3.5025799450779));
#28676=CARTESIAN_POINT('Ctrl Pts',(0.0840465917532045,-0.127640331046499,
3.49728682502665));
#28677=CARTESIAN_POINT('Ctrl Pts',(0.0374537582415282,-0.140096572423083,
3.49464026500102));
#28678=CARTESIAN_POINT('Ctrl Pts',(0.116913659442511,0.100696009035912,
4.01607920499693));
#28679=CARTESIAN_POINT('Ctrl Pts',(0.15040278985558,0.0618132685417683,
4.01343264497131));
#28680=CARTESIAN_POINT('Ctrl Pts',(0.17494437076274,-0.0513331417022419,
4.00813952492005));
#28681=CARTESIAN_POINT('Ctrl Pts',(0.0515151396231945,-0.17507865733575,
4.00019984484318));
#28682=CARTESIAN_POINT('Ctrl Pts',(-0.119076904876771,-0.138089613969001,
3.9922601647663));
#28683=CARTESIAN_POINT('Ctrl Pts',(-0.180643768642924,0.0251157894691961,
3.98432048468943));
#28684=CARTESIAN_POINT('Ctrl Pts',(-0.0768181153328184,0.165435267997838,
3.97638080461255));
#28685=CARTESIAN_POINT('Ctrl Pts',(0.0973408978391562,0.154229954870798,
3.96844112453568));
#28686=CARTESIAN_POINT('Ctrl Pts',(0.182376570303567,0.00184388772387479,
3.9605014444588));
#28687=CARTESIAN_POINT('Ctrl Pts',(0.100432518024861,-0.152245093163996,
3.95256176438192));
#28688=CARTESIAN_POINT('Ctrl Pts',(-0.0734653243360244,-0.166934402953208,
3.94462208430505));
#28689=CARTESIAN_POINT('Ctrl Pts',(-0.180099955267235,-0.0287862227331087,
3.93668240422817));
#28690=CARTESIAN_POINT('Ctrl Pts',(-0.121839177317157,0.135719942641123,
3.9287427241513));
#28691=CARTESIAN_POINT('Ctrl Pts',(0.0479747894892283,0.175963002958517,
3.92080304407442));
#28692=CARTESIAN_POINT('Ctrl Pts',(0.173864125597012,0.0550988560374321,
3.91286336399754));
#28693=CARTESIAN_POINT('Ctrl Pts',(0.140567423109983,-0.116212816074597,
3.90492368392067));
#28694=CARTESIAN_POINT('Ctrl Pts',(-0.0214296173447312,-0.181122539961793,
3.89698400384379));
#28695=CARTESIAN_POINT('Ctrl Pts',(-0.163806186794094,-0.0802006535492451,
3.88904432376692));
#28696=CARTESIAN_POINT('Ctrl Pts',(-0.156205535929391,0.0941511635800416,
3.88110464369004));
#28697=CARTESIAN_POINT('Ctrl Pts',(-0.005586647457645,0.182300297549597,
3.87316496361317));
#28698=CARTESIAN_POINT('Ctrl Pts',(0.150147248343024,0.103539432915148,
3.86522528353629));
#28699=CARTESIAN_POINT('Ctrl Pts',(0.168409737102627,-0.0700197873807462,
3.85728560345941));
#28700=CARTESIAN_POINT('Ctrl Pts',(0.0324800992415292,-0.179470479754251,
3.84934592338254));
#28701=CARTESIAN_POINT('Ctrl Pts',(-0.133187579060394,-0.124602082269994,
3.84140624330566));
#28702=CARTESIAN_POINT('Ctrl Pts',(-0.17691173791599,0.0443491496337192,
3.83346656322879));
#28703=CARTESIAN_POINT('Ctrl Pts',(-0.0586595315107243,0.172695308053416,
3.82552688315191));
#28704=CARTESIAN_POINT('Ctrl Pts',(0.113300008356683,0.142925568707939,
3.81758720307504));
#28705=CARTESIAN_POINT('Ctrl Pts',(0.181524636378177,-0.0177035721096275,
3.80964752299816));
#28706=CARTESIAN_POINT('Ctrl Pts',(0.0835494341804624,-0.162123724738966,
3.80170784292129));
#28707=CARTESIAN_POINT('Ctrl Pts',(-0.0909217305086156,-0.158107080801413,
3.7937681628444));
#28708=CARTESIAN_POINT('Ctrl Pts',(-0.18214702579272,-0.00933118813597588,
3.78582848276753));
#28709=CARTESIAN_POINT('Ctrl Pts',(-0.106602645259627,0.147988128242044,
3.77788880269065));
#28710=CARTESIAN_POINT('Ctrl Pts',(0.0665446937287967,0.169812878822259,
3.76994912261378));
#28711=CARTESIAN_POINT('Ctrl Pts',(0.178765223990991,0.0361608181406009,
3.7620094425369));
#28712=CARTESIAN_POINT('Ctrl Pts',(0.127312379282745,-0.130599265535886,
3.75406976246003));
#28713=CARTESIAN_POINT('Ctrl Pts',(-0.0407047855299705,-0.177785630781348,
3.74613008238315));
#28714=CARTESIAN_POINT('Ctrl Pts',(-0.171453574108382,-0.0621955143269609,
3.73819040230628));
#28715=CARTESIAN_POINT('Ctrl Pts',(-0.145223368124595,0.110339401066487,
3.7302507222294));
#28716=CARTESIAN_POINT('Ctrl Pts',(0.0139700521550768,0.18185006934563,
3.72231104215253));
#28717=CARTESIAN_POINT('Ctrl Pts',(0.160372810275332,0.0868629483698537,
3.71437136207565));
#28718=CARTESIAN_POINT('Ctrl Pts',(0.15994186929589,-0.087653913339944,
3.70643168199877));
#28719=CARTESIAN_POINT('Ctrl Pts',(0.013071788942189,-0.181916844788939,
3.6984920019219));
#28720=CARTESIAN_POINT('Ctrl Pts',(-0.145766524138762,-0.109620848843756,
3.69055232184502));
#28721=CARTESIAN_POINT('Ctrl Pts',(-0.171144321725171,0.06304150400269,
3.68261264176815));
#28722=CARTESIAN_POINT('Ctrl Pts',(-0.039826269011209,0.177984489264188,
3.67467296169127));
#28723=CARTESIAN_POINT('Ctrl Pts',(0.127955809817362,0.129968921992697,
3.66673328161439));
#28724=CARTESIAN_POINT('Ctrl Pts',(0.178584458888466,-0.0370432344610292,
3.65879360153752));
#28725=CARTESIAN_POINT('Ctrl Pts',(0.0657052360091523,-0.170139449612234,
3.65085392146064));
#28726=CARTESIAN_POINT('Ctrl Pts',(-0.107332204463161,-0.147459848777779,
3.64291424138377));
#28727=CARTESIAN_POINT('Ctrl Pts',(-0.182098723988745,0.0102306295082514,
3.63497456130689));
#28728=CARTESIAN_POINT('Ctrl Pts',(-0.0901397813258339,0.158554191001936,
3.62703488123002));
#28729=CARTESIAN_POINT('Ctrl Pts',(0.0843490755327352,0.161709110561297,
3.61909520115314));
#28730=CARTESIAN_POINT('Ctrl Pts',(0.181609876119891,0.0168069020193158,
3.61115552107626));
#28731=CARTESIAN_POINT('Ctrl Pts',(0.11259272547993,-0.14348343554309,3.60321584099938));
#28732=CARTESIAN_POINT('Ctrl Pts',(-0.0595116136917225,-0.1724033835878,
3.59527616092251));
#28733=CARTESIAN_POINT('Ctrl Pts',(-0.17712876751773,-0.0434751386137106,
3.58733648084563));
#28734=CARTESIAN_POINT('Ctrl Pts',(-0.132570272379398,0.125258785670915,
3.57939680076876));
#28735=CARTESIAN_POINT('Ctrl Pts',(0.0333654249967142,0.179306991453011,
3.57145712069188));
#28736=CARTESIAN_POINT('Ctrl Pts',(0.16875469474836,0.0691889591605158,
3.56351744061501));
#28737=CARTESIAN_POINT('Ctrl Pts',(0.149631713131164,-0.104283094234219,
3.55557776053813));
#28738=CARTESIAN_POINT('Ctrl Pts',(-0.00648228852693025,-0.182263845309582,
3.54763808046125));
#28739=CARTESIAN_POINT('Ctrl Pts',(-0.156677605505559,-0.0933915342729034,
3.53969840038438));
#28740=CARTESIAN_POINT('Ctrl Pts',(-0.163390540317638,0.0810339766078996,
3.5317587203075));
#28741=CARTESIAN_POINT('Ctrl Pts',(-0.0205691901156568,0.181176596665036,
3.52381904023063));
#28742=CARTESIAN_POINT('Ctrl Pts',(0.141207069227503,0.115615351338242,
3.51587936015375));
#28743=CARTESIAN_POINT('Ctrl Pts',(0.173454096992073,-0.0561631599472297,
3.50793968007688));
#28744=CARTESIAN_POINT('Ctrl Pts',(0.089426887306191,-0.135811307301286,
3.50264656002563));
#28745=CARTESIAN_POINT('Ctrl Pts',(0.0398513841857336,-0.149064942821849,
3.5));
#28746=CARTESIAN_POINT('Ctrl Pts',(0.095811615272233,0.0825211298936557,
4.));
#28747=CARTESIAN_POINT('Ctrl Pts',(0.102493030557671,0.0762815759767258,
4.));
#28748=CARTESIAN_POINT('Ctrl Pts',(0.10839405706188,0.0693097484661253,
4.));
#28749=CARTESIAN_POINT('Ctrl Pts',(0.11350885289652,0.0617853075148104,
4.));
#28750=CARTESIAN_POINT('Ctrl Pts',(0.117424080053794,0.0560255672420171,
4.));
#28751=CARTESIAN_POINT('Ctrl Pts',(0.120878299816185,0.0499406938168944,
4.));
#28752=CARTESIAN_POINT('Ctrl Pts',(0.123857056765335,0.0435961076613069,
4.));
#28753=CARTESIAN_POINT('Ctrl Pts',(0.125170781948423,0.0407979462969676,
4.));
#28754=CARTESIAN_POINT('Ctrl Pts',(0.126390002992329,0.0379525898756446,
4.));
#28755=CARTESIAN_POINT('Ctrl Pts',(0.12751038950843,0.0350750832122783,
4.));
#28756=CARTESIAN_POINT('Ctrl Pts',(0.131085166597008,0.0258939258664803,
4.));
#28757=CARTESIAN_POINT('Ctrl Pts',(0.133669431833427,0.0163619242015854,
4.));
#28758=CARTESIAN_POINT('Ctrl Pts',(0.135230958047781,0.0066616777752228,
4.));
#28759=CARTESIAN_POINT('Ctrl Pts',(0.135923073683569,0.00236223524203686,
4.));
#28760=CARTESIAN_POINT('Ctrl Pts',(0.136413711726375,-0.0019706858607116,
4.));
#28761=CARTESIAN_POINT('Ctrl Pts',(0.136697089502038,-0.00632254181082518,
4.));
#28762=CARTESIAN_POINT('Ctrl Pts',(0.136879678085431,-0.00912656979504798,
4.));
#28763=CARTESIAN_POINT('Ctrl Pts',(0.136975856810266,-0.011936494905405,
4.));
#28764=CARTESIAN_POINT('Ctrl Pts',(0.136984537674321,-0.0147391030393356,
4.));
#28765=CARTESIAN_POINT('Ctrl Pts',(0.137010531466213,-0.0231311723225325,
4.));
#28766=CARTESIAN_POINT('Ctrl Pts',(0.136255503035819,-0.0314800211532621,
4.));
#28767=CARTESIAN_POINT('Ctrl Pts',(0.134693290097439,-0.0396806821547801,
4.));
#28768=CARTESIAN_POINT('Ctrl Pts',(0.133704762250079,-0.0448698478361003,
4.));
#28769=CARTESIAN_POINT('Ctrl Pts',(0.132392592878428,-0.0499999054788172,
4.));
#28770=CARTESIAN_POINT('Ctrl Pts',(0.130776991260223,-0.0550529928649125,
4.));
#28771=CARTESIAN_POINT('Ctrl Pts',(0.129445892801333,-0.0592162449664668,
4.));
#28772=CARTESIAN_POINT('Ctrl Pts',(0.127906314848104,-0.0633316423760335,
4.));
#28773=CARTESIAN_POINT('Ctrl Pts',(0.126180878863323,-0.0673610722009708,
4.));
#28774=CARTESIAN_POINT('Ctrl Pts',(0.122312843187174,-0.0763941388895448,
4.));
#28775=CARTESIAN_POINT('Ctrl Pts',(0.117508253438465,-0.0850205194401279,
4.));
#28776=CARTESIAN_POINT('Ctrl Pts',(0.111900166266883,-0.0931314900308112,
4.));
#28777=CARTESIAN_POINT('Ctrl Pts',(0.108605841530307,-0.097896068439994,
4.));
#28778=CARTESIAN_POINT('Ctrl Pts',(0.105033346987346,-0.102482765945667,
4.));
#28779=CARTESIAN_POINT('Ctrl Pts',(0.101203104491781,-0.106867390005116,
4.));
#28780=CARTESIAN_POINT('Ctrl Pts',(0.0988795404734533,-0.109527261987172,
4.));
#28781=CARTESIAN_POINT('Ctrl Pts',(0.0964620699804362,-0.112111128650417,
4.));
#28782=CARTESIAN_POINT('Ctrl Pts',(0.0939639375491823,-0.114605366763082,
4.));
#28783=CARTESIAN_POINT('Ctrl Pts',(0.0874788757256353,-0.121080319075824,
4.));
#28784=CARTESIAN_POINT('Ctrl Pts',(0.0804377540716352,-0.126968968726175,
4.));
#28785=CARTESIAN_POINT('Ctrl Pts',(0.0729230547225638,-0.132178932127324,
4.));
#28786=CARTESIAN_POINT('Ctrl Pts',(0.0694491809116136,-0.134587379168854,
4.));
#28787=CARTESIAN_POINT('Ctrl Pts',(0.0658808132415588,-0.136845565695848,
4.));
#28788=CARTESIAN_POINT('Ctrl Pts',(0.0622290543017492,-0.138943290379685,
4.));
#28789=CARTESIAN_POINT('Ctrl Pts',(0.0562216582547972,-0.142394192583524,
4.));
#28790=CARTESIAN_POINT('Ctrl Pts',(0.0499865922958981,-0.145412833318798,
4.));
#28791=CARTESIAN_POINT('Ctrl Pts',(0.0435567401413007,-0.147956905966761,
4.));
#28792=CARTESIAN_POINT('Ctrl Pts',(0.0423577886630555,-0.148431290072134,
4.));
#28793=CARTESIAN_POINT('Ctrl Pts',(0.0411520494229064,-0.148889152887265,
4.));
#28794=CARTESIAN_POINT('Ctrl Pts',(0.0399398308045252,-0.149330586455588,
4.));
#28795=CARTESIAN_POINT('Ctrl Pts',(-0.126543984365092,-0.000100563349596846,
3.91934196736194));
#28796=CARTESIAN_POINT('Ctrl Pts',(-0.126601870201444,-0.00676638730964717,
3.91976237798504));
#28797=CARTESIAN_POINT('Ctrl Pts',(-0.126120638953643,-0.0134238307402375,
3.92018278860814));
#28798=CARTESIAN_POINT('Ctrl Pts',(-0.125071086204593,-0.0199904298605203,
3.92060319923124));
#28799=CARTESIAN_POINT('Ctrl Pts',(-0.118463964029756,-0.0613283451774388,
3.92324975925687));
#28800=CARTESIAN_POINT('Ctrl Pts',(-0.089334672430595,-0.0990661662809851,
3.92589631928249));
#28801=CARTESIAN_POINT('Ctrl Pts',(-0.0510182636513927,-0.115928743690777,
3.92854287930812));
#28802=CARTESIAN_POINT('Ctrl Pts',(-0.0127018548721904,-0.132791321100569,
3.93118943933374));
#28803=CARTESIAN_POINT('Ctrl Pts',(0.0348016710870533,-0.128778654816608,
3.93383599935937));
#28804=CARTESIAN_POINT('Ctrl Pts',(0.0697457276620979,-0.10572614363048,
3.93648255938499));
#28805=CARTESIAN_POINT('Ctrl Pts',(0.104689784237142,-0.0826736324443521,
3.93912911941062));
#28806=CARTESIAN_POINT('Ctrl Pts',(0.127074371427988,-0.0405812763560585,
3.94177567943624));
#28807=CARTESIAN_POINT('Ctrl Pts',(0.126652103797309,0.00127848798181101,
3.94442223946187));
#28808=CARTESIAN_POINT('Ctrl Pts',(0.126229836166631,0.0431382523196808,
3.94706879948749));
#28809=CARTESIAN_POINT('Ctrl Pts',(0.103000713714428,0.0847654249071265,
3.94971535951312));
#28810=CARTESIAN_POINT('Ctrl Pts',(0.067598717604338,0.107109484137676,
3.95236191953875));
#28811=CARTESIAN_POINT('Ctrl Pts',(0.0321967214942486,0.129453543368225,
3.95500847956437));
#28812=CARTESIAN_POINT('Ctrl Pts',(-0.0153781482737276,0.132514489241879,
3.95765503958999));
#28813=CARTESIAN_POINT('Ctrl Pts',(-0.0533465659413221,0.114879485769171,
3.96030159961562));
#28814=CARTESIAN_POINT('Ctrl Pts',(-0.0913149836089167,0.0972444822964635,
3.96294815964124));
#28815=CARTESIAN_POINT('Ctrl Pts',(-0.11967694917613,0.0589135294773952,
3.96559471966687));
#28816=CARTESIAN_POINT('Ctrl Pts',(-0.12544884800723,0.0174567123195785,
3.9682412796925));
#28817=CARTESIAN_POINT('Ctrl Pts',(-0.1262490134813,0.0117095024801126,
3.96860817558231));
#28818=CARTESIAN_POINT('Ctrl Pts',(-0.126615029050668,0.00590221784225734,
3.96897507147213));
#28819=CARTESIAN_POINT('Ctrl Pts',(-0.126567406925801,8.9117089303592E-5,
3.96934196736194));
#28820=CARTESIAN_POINT('Ctrl Pts',(-0.0398513841857263,-0.149064942821851,
4.));
#28821=CARTESIAN_POINT('Ctrl Pts',(-0.0894268873061843,-0.13581130730129,
3.99735343997437));
#28822=CARTESIAN_POINT('Ctrl Pts',(-0.173454116750112,-0.0561632816072737,
3.99206031992313));
#28823=CARTESIAN_POINT('Ctrl Pts',(-0.141207051852386,0.115615412698802,
3.98412063984625));
#28824=CARTESIAN_POINT('Ctrl Pts',(0.0205691872966891,0.181176549232701,
3.97618095976937));
#28825=CARTESIAN_POINT('Ctrl Pts',(0.16339053139201,0.0810339956098913,
3.9682412796925));
#28826=CARTESIAN_POINT('Ctrl Pts',(0.156677599794682,-0.0933915431448235,
3.96030159961562));
#28827=CARTESIAN_POINT('Ctrl Pts',(0.00648228676056323,-0.182263829019595,
3.95236191953875));
#28828=CARTESIAN_POINT('Ctrl Pts',(-0.149631704989928,-0.104283093629962,
3.94442223946187));
#28829=CARTESIAN_POINT('Ctrl Pts',(-0.168754687429674,0.0691889583215889,
3.93648255938499));
#28830=CARTESIAN_POINT('Ctrl Pts',(-0.0333654229848094,0.179306981584077,
3.92854287930812));
#28831=CARTESIAN_POINT('Ctrl Pts',(0.132570265831228,0.125258780485074,
3.92060319923124));
#28832=CARTESIAN_POINT('Ctrl Pts',(0.17712875926901,-0.0434751369680033,
3.91266351915436));
#28833=CARTESIAN_POINT('Ctrl Pts',(0.059511610779771,-0.172403375181386,
3.90472383907749));
#28834=CARTESIAN_POINT('Ctrl Pts',(-0.112592720088119,-0.143483428861666,
3.89678415900062));
#28835=CARTESIAN_POINT('Ctrl Pts',(-0.181609867534042,0.0168069012899025,
3.88884447892373));
#28836=CARTESIAN_POINT('Ctrl Pts',(-0.0843490715154628,0.161709102853824,
3.88090479884686));
#28837=CARTESIAN_POINT('Ctrl Pts',(0.0901397770410241,0.158554183500776,
3.87296511876998));
#28838=CARTESIAN_POINT('Ctrl Pts',(0.182098715355847,0.0102306290122647,
3.86502543869311));
#28839=CARTESIAN_POINT('Ctrl Pts',(0.107332199369115,-0.147459841777235,
3.85708575861623));
#28840=CARTESIAN_POINT('Ctrl Pts',(-0.0657052328909015,-0.17013944154474,
3.84914607853936));
#28841=CARTESIAN_POINT('Ctrl Pts',(-0.178584450418103,-0.0370432327022405,
3.84120639846248));
#28842=CARTESIAN_POINT('Ctrl Pts',(-0.127955803747328,0.129968915826709,
3.83326671838561));
#28843=CARTESIAN_POINT('Ctrl Pts',(0.039826267121788,0.177984480821945,
3.82532703830873));
#28844=CARTESIAN_POINT('Ctrl Pts',(0.171144313607041,0.063041501012073,
3.81738735823185));
#28845=CARTESIAN_POINT('Ctrl Pts',(0.145766517224248,-0.109620843643728,
3.80944767815498));
#28846=CARTESIAN_POINT('Ctrl Pts',(-0.0130717883220708,-0.181916836159762,
3.8015079980781));
#28847=CARTESIAN_POINT('Ctrl Pts',(-0.159941861709037,-0.0876539091820477,
3.79356831800123));
#28848=CARTESIAN_POINT('Ctrl Pts',(-0.160372802668024,0.0868629442494614,
3.78562863792435));
#28849=CARTESIAN_POINT('Ctrl Pts',(-0.013970051492431,0.181850060719556,
3.77768895784748));
#28850=CARTESIAN_POINT('Ctrl Pts',(0.145223361235896,0.110339395832533,
3.7697492777706));
#28851=CARTESIAN_POINT('Ctrl Pts',(0.171453565975463,-0.0621955113766863,
3.76180959769372));
#28852=CARTESIAN_POINT('Ctrl Pts',(0.0407047835991549,-0.177785622348059,
3.75386991761685));
#28853=CARTESIAN_POINT('Ctrl Pts',(-0.127312373243651,-0.130599259340906,
3.74593023753997));
#28854=CARTESIAN_POINT('Ctrl Pts',(-0.178765215511242,0.0361608164252855,
3.7379905574631));
#28855=CARTESIAN_POINT('Ctrl Pts',(-0.0665446905722607,0.169812870767156,
3.73005087738622));
#28856=CARTESIAN_POINT('Ctrl Pts',(0.106602640202898,0.147988121222216,
3.72211119730934));
#28857=CARTESIAN_POINT('Ctrl Pts',(0.182147017152552,-0.0093311876933208,
3.71417151723247));
#28858=CARTESIAN_POINT('Ctrl Pts',(0.0909217261957518,-0.158107073301583,
3.70623183715559));
#28859=CARTESIAN_POINT('Ctrl Pts',(-0.0835494302172658,-0.162123717048593,
3.69829215707872));
#28860=CARTESIAN_POINT('Ctrl Pts',(-0.181524627767524,-0.0177035712699219,
3.69035247700185));
#28861=CARTESIAN_POINT('Ctrl Pts',(-0.113300002982309,0.14292556192831,
3.68241279692496));
#28862=CARTESIAN_POINT('Ctrl Pts',(0.0586595287281965,0.172695299861449,
3.67447311684809));
#28863=CARTESIAN_POINT('Ctrl Pts',(0.176911729524118,0.0443491475303153,
3.66653343677121));
#28864=CARTESIAN_POINT('Ctrl Pts',(0.133187572742707,-0.124602076359984,
3.65859375669434));
#28865=CARTESIAN_POINT('Ctrl Pts',(-0.0324800977009374,-0.179470471240069,
3.65065407661746));
#28866=CARTESIAN_POINT('Ctrl Pts',(-0.168409729113823,-0.0700197840611982,
3.64271439654059));
#28867=CARTESIAN_POINT('Ctrl Pts',(-0.150147241221285,0.103539428007117,
3.63477471646371));
#28868=CARTESIAN_POINT('Ctrl Pts',(0.00558664719359638,0.182300288895857,
3.62683503638684));
#28869=CARTESIAN_POINT('Ctrl Pts',(0.156205528517827,0.094151159125646,
3.61889535630996));
#28870=CARTESIAN_POINT('Ctrl Pts',(0.163806179027695,-0.0802006497663837,
3.61095567623308));
#28871=CARTESIAN_POINT('Ctrl Pts',(0.0214296163208854,-0.181122531330724,
3.60301599615621));
#28872=CARTESIAN_POINT('Ctrl Pts',(-0.140567416427732,-0.116212810634341,
3.59507631607934));
#28873=CARTESIAN_POINT('Ctrl Pts',(-0.173864117377934,0.0550988535555318,
3.58713663600245));
#28874=CARTESIAN_POINT('Ctrl Pts',(-0.0479747871584019,0.175962994372803,
3.57919695592558));
#28875=CARTESIAN_POINT('Ctrl Pts',(0.121839171429706,0.13571993663382,3.5712572758487));
#28876=CARTESIAN_POINT('Ctrl Pts',(0.180099946935509,-0.0287862221383337,
3.56331759577183));
#28877=CARTESIAN_POINT('Ctrl Pts',(0.0734653204375665,-0.166934393666355,
3.55537791569495));
#28878=CARTESIAN_POINT('Ctrl Pts',(-0.100432512451176,-0.152245088347237,
3.54743823561807));
#28879=CARTESIAN_POINT('Ctrl Pts',(-0.182376563237206,0.00184389181179004,
3.5394985555412));
#28880=CARTESIAN_POINT('Ctrl Pts',(-0.0973408901199132,0.154229940417525,
3.53155887546432));
#28881=CARTESIAN_POINT('Ctrl Pts',(0.0768181056158631,0.16543527210962,
3.52361919538745));
#28882=CARTESIAN_POINT('Ctrl Pts',(0.180643771975638,0.0251157687415861,
3.51567951531057));
#28883=CARTESIAN_POINT('Ctrl Pts',(0.11907687582224,-0.13808957637103,3.50773983523369));
#28884=CARTESIAN_POINT('Ctrl Pts',(-0.0515150906951779,-0.17507869823889,
3.49980015515682));
#28885=CARTESIAN_POINT('Ctrl Pts',(-0.174944455635001,-0.0513330523253054,
3.49186047507995));
#28886=CARTESIAN_POINT('Ctrl Pts',(-0.15040278985559,0.061813268541742,
3.4865673550287));
#28887=CARTESIAN_POINT('Ctrl Pts',(-0.116913659442529,0.100696009035892,
3.48392079500307));
#28888=CARTESIAN_POINT('Ctrl Pts',(-0.0374537582415214,-0.140096572423085,
4.00535973499898));
#28889=CARTESIAN_POINT('Ctrl Pts',(-0.0840465917531983,-0.127640331046503,
4.00271317497335));
#28890=CARTESIAN_POINT('Ctrl Pts',(-0.163018391644278,-0.0527842636924701,
3.9974200549221));
#28891=CARTESIAN_POINT('Ctrl Pts',(-0.132711445038627,0.108659505929172,
3.98948037484522));
#28892=CARTESIAN_POINT('Ctrl Pts',(0.0193316589618159,0.170276210290963,
3.98154069476835));
#28893=CARTESIAN_POINT('Ctrl Pts',(0.153560273670542,0.0761586515231869,
3.97360101469147));
#28894=CARTESIAN_POINT('Ctrl Pts',(0.147251220113796,-0.0877727173150906,
3.9656613346146));
#28895=CARTESIAN_POINT('Ctrl Pts',(0.00609228527799324,-0.171298074778515,
3.95772165453772));
#28896=CARTESIAN_POINT('Ctrl Pts',(-0.140629235808745,-0.0980089865709976,
3.94978197446085));
#28897=CARTESIAN_POINT('Ctrl Pts',(-0.158601699646316,0.0650262612179893,
3.94184229438397));
#28898=CARTESIAN_POINT('Ctrl Pts',(-0.0313580195928739,0.168519123651227,
3.93390261430709));
#28899=CARTESIAN_POINT('Ctrl Pts',(0.124594284186381,0.117722688377688,
3.92596293423022));
#28900=CARTESIAN_POINT('Ctrl Pts',(0.166471952300676,-0.0408594909006909,
3.91802325415334));
#28901=CARTESIAN_POINT('Ctrl Pts',(0.0559311433781364,-0.162030867082874,
3.91008357407647));
#28902=CARTESIAN_POINT('Ctrl Pts',(-0.105818671147842,-0.134850865686472,
3.90214389399959));
#28903=CARTESIAN_POINT('Ctrl Pts',(-0.170683458351015,0.0157957278163147,
3.89420421392272));
#28904=CARTESIAN_POINT('Ctrl Pts',(-0.0792742785975418,0.151980006905501,
3.88626453384583));
#28905=CARTESIAN_POINT('Ctrl Pts',(0.0847165910600508,0.149014900695642,
3.87832485376897));
#28906=CARTESIAN_POINT('Ctrl Pts',(0.171142895043338,0.00961511158303258,
3.87038517369209));
#28907=CARTESIAN_POINT('Ctrl Pts',(0.100874645356521,-0.138588040970374,
3.86244549361521));
#28908=CARTESIAN_POINT('Ctrl Pts',(-0.0617521312792973,-0.159903141162322,
3.85450581353833));
#28909=CARTESIAN_POINT('Ctrl Pts',(-0.16784006298206,-0.0348145568958948,
3.84656613346146));
#28910=CARTESIAN_POINT('Ctrl Pts',(-0.120257447440646,0.122149442277835,
3.83862645338458));
#28911=CARTESIAN_POINT('Ctrl Pts',(0.0374301523251976,0.167276190066077,
3.83068677330771));
#28912=CARTESIAN_POINT('Ctrl Pts',(0.16084755591865,0.0592486606509017,
3.82274709323083));
#28913=CARTESIAN_POINT('Ctrl Pts',(0.136996593904535,-0.103025595219711,
3.81480741315396));
#28914=CARTESIAN_POINT('Ctrl Pts',(-0.0122853348660984,-0.170971958460368,
3.80686773307708));
#28915=CARTESIAN_POINT('Ctrl Pts',(-0.150319090379167,-0.0823802834081873,
3.7989280530002));
#28916=CARTESIAN_POINT('Ctrl Pts',(-0.150724104127725,0.0816369062340208,
3.79098837292333));
#28917=CARTESIAN_POINT('Ctrl Pts',(-0.0131295547672976,0.170909200509922,
3.78304869284645));
#28918=CARTESIAN_POINT('Ctrl Pts',(0.136486116452099,0.103700916303616,
3.77510901276958));
#28919=CARTESIAN_POINT('Ctrl Pts',(0.161138202371193,-0.0584535692901865,
3.7671693326927));
#28920=CARTESIAN_POINT('Ctrl Pts',(0.0382558135770412,-0.167089295749672,
3.75922965261583));
#28921=CARTESIAN_POINT('Ctrl Pts',(-0.119652728407108,-0.122741861689914,
3.75128997253895));
#28922=CARTESIAN_POINT('Ctrl Pts',(-0.168009952491177,0.0339852304727166,
3.74335029246208));
#28923=CARTESIAN_POINT('Ctrl Pts',(-0.0625410836756577,0.159596218248545,
3.73541061238519));
#28924=CARTESIAN_POINT('Ctrl Pts',(0.100188979521,0.139084536914507,3.72747093230832));
#28925=CARTESIAN_POINT('Ctrl Pts',(0.171188290801939,-0.00876978441559563,
3.71953125223144));
#28926=CARTESIAN_POINT('Ctrl Pts',(0.0854514948832616,-0.148594690515994,
3.71159157215457));
#28927=CARTESIAN_POINT('Ctrl Pts',(-0.078522747064207,-0.15236967617626,
3.7036518920777));
#28928=CARTESIAN_POINT('Ctrl Pts',(-0.170603346965352,-0.0166384503801673,
3.69571221200081));
#28929=CARTESIAN_POINT('Ctrl Pts',(-0.106483400945028,0.134326562361009,
3.68777253192394));
#28930=CARTESIAN_POINT('Ctrl Pts',(0.0551303261464719,0.162305228353258,
3.67983285184707));
#28931=CARTESIAN_POINT('Ctrl Pts',(0.166267979972926,0.0416809173321745,
3.67189317177019));
#28932=CARTESIAN_POINT('Ctrl Pts',(0.125174451332285,-0.117105494319316,
3.66395349169331));
#28933=CARTESIAN_POINT('Ctrl Pts',(-0.030525959180801,-0.168672777085747,
3.65601381161644));
#28934=CARTESIAN_POINT('Ctrl Pts',(-0.158277495465476,-0.0658071010063173,
3.64807413153956));
#28935=CARTESIAN_POINT('Ctrl Pts',(-0.141113755224281,0.0973100629822772,
3.64013445146269));
#28936=CARTESIAN_POINT('Ctrl Pts',(0.0052505311332342,0.171332341076135,
3.63219477138581));
#28937=CARTESIAN_POINT('Ctrl Pts',(0.146807550619315,0.0884866316215429,
3.62425509130893));
#28938=CARTESIAN_POINT('Ctrl Pts',(0.153950914206089,-0.0753754432509509,
3.61631541123206));
#28939=CARTESIAN_POINT('Ctrl Pts',(0.0201403209773194,-0.170225442331889,
3.60837573115518));
#28940=CARTESIAN_POINT('Ctrl Pts',(-0.132110292756286,-0.109220961906395,
3.60043605107832));
#28941=CARTESIAN_POINT('Ctrl Pts',(-0.163403724919573,0.0517838760841091,
3.59249637100142));
#28942=CARTESIAN_POINT('Ctrl Pts',(-0.0450884233166185,0.165376324696236,
3.58455669092456));
#28943=CARTESIAN_POINT('Ctrl Pts',(0.114508817305019,0.12755445762053,3.57661701084768));
#28944=CARTESIAN_POINT('Ctrl Pts',(0.169264380890674,-0.0270543226210457,
3.56867733077081));
#28945=CARTESIAN_POINT('Ctrl Pts',(0.0690453395039173,-0.156890922368865,
3.56073765069393));
#28946=CARTESIAN_POINT('Ctrl Pts',(-0.0943900724603247,-0.14308538709325,
3.55279797061705));
#28947=CARTESIAN_POINT('Ctrl Pts',(-0.171404026434103,0.00173295556863096,
3.54485829054018));
#28948=CARTESIAN_POINT('Ctrl Pts',(-0.0914844550586914,0.144950822161685,
3.5369186104633));
#28949=CARTESIAN_POINT('Ctrl Pts',(0.0721964071034376,0.155481994234803,
3.52897893038643));
#28950=CARTESIAN_POINT('Ctrl Pts',(0.169775487141934,0.0236046990516893,
3.52103925030955));
#28951=CARTESIAN_POINT('Ctrl Pts',(0.111912712954128,-0.129781529920537,
3.51309957023267));
#28952=CARTESIAN_POINT('Ctrl Pts',(-0.0484157273859087,-0.164545231516157,
3.5051598901558));
#28953=CARTESIAN_POINT('Ctrl Pts',(-0.164419065508765,-0.0482446412057121,
3.49722021007893));
#28954=CARTESIAN_POINT('Ctrl Pts',(-0.141353928983959,0.0580943237828579,
3.49192709002767));
#28955=CARTESIAN_POINT('Ctrl Pts',(-0.109879644719102,0.094637715988474,
3.48928053000205));
#28956=CARTESIAN_POINT('Ctrl Pts',(-0.0350561322973164,-0.13112820202432,
4.01071946999795));
#28957=CARTESIAN_POINT('Ctrl Pts',(-0.0786662962002123,-0.119469354791716,
4.00807290997233));
#28958=CARTESIAN_POINT('Ctrl Pts',(-0.152582666538444,-0.0494052457776665,
4.00277978992108));
#28959=CARTESIAN_POINT('Ctrl Pts',(-0.124215838224868,0.101703599159542,
3.9948401098442));
#28960=CARTESIAN_POINT('Ctrl Pts',(0.0180941306269427,0.159375871349225,
3.98690042976732));
#28961=CARTESIAN_POINT('Ctrl Pts',(0.143730015949074,0.0712833074364824,
3.97896074969045));
#28962=CARTESIAN_POINT('Ctrl Pts',(0.137824840432911,-0.0821538914853577,
3.97102106961357));
#28963=CARTESIAN_POINT('Ctrl Pts',(0.0057022837954231,-0.160332320537436,
3.9630813895367));
#28964=CARTESIAN_POINT('Ctrl Pts',(-0.131626766627563,-0.0917348795120337,
3.95514170945982));
#28965=CARTESIAN_POINT('Ctrl Pts',(-0.148448711862958,0.0608635641143897,
3.94720202938295));
#28966=CARTESIAN_POINT('Ctrl Pts',(-0.0293506162009384,0.157731265718376,
3.93926234930607));
#28967=CARTESIAN_POINT('Ctrl Pts',(0.116618302541534,0.110186596270301,
3.93132266922919));
#28968=CARTESIAN_POINT('Ctrl Pts',(0.155815145332341,-0.0382438448333786,
3.92338298915232));
#28969=CARTESIAN_POINT('Ctrl Pts',(0.0523506759765019,-0.151658358984361,
3.91544330907544));
#28970=CARTESIAN_POINT('Ctrl Pts',(-0.0990446222075651,-0.126218302511277,
3.90750362899857));
#28971=CARTESIAN_POINT('Ctrl Pts',(-0.159757049167988,0.0147845543427269,
3.89956394892169));
#28972=CARTESIAN_POINT('Ctrl Pts',(-0.0741994856796208,0.142250910957177,
3.89162426884482));
#28973=CARTESIAN_POINT('Ctrl Pts',(0.0792934050790776,0.139475617890508,
3.88368458876794));
#28974=CARTESIAN_POINT('Ctrl Pts',(0.160187074730829,0.0089995941538004,
3.87574490869107));
#28975=CARTESIAN_POINT('Ctrl Pts',(0.0944170913439271,-0.129716240163513,
3.86780522861419));
#28976=CARTESIAN_POINT('Ctrl Pts',(-0.0577990296676931,-0.149666840779905,
3.85986554853731));
#28977=CARTESIAN_POINT('Ctrl Pts',(-0.157095675546018,-0.0325858810895492,
3.85192586846044));
#28978=CARTESIAN_POINT('Ctrl Pts',(-0.112559091133964,0.114329968728961,
3.84398618838356));
#28979=CARTESIAN_POINT('Ctrl Pts',(0.0350340375286068,0.156567899310209,
3.83604650830669));
#28980=CARTESIAN_POINT('Ctrl Pts',(0.150550798230259,0.0554558202897304,
3.8281068282298));
#28981=CARTESIAN_POINT('Ctrl Pts',(0.128226670584821,-0.0964303467956928,
3.82016714815294));
#28982=CARTESIAN_POINT('Ctrl Pts',(-0.0114988814101258,-0.160027080760974,
3.81222746807605));
#28983=CARTESIAN_POINT('Ctrl Pts',(-0.140696319049298,-0.0771066576343268,
3.80428778799918));
#28984=CARTESIAN_POINT('Ctrl Pts',(-0.141075405587426,0.0764108682185801,
3.79634810792231));
#28985=CARTESIAN_POINT('Ctrl Pts',(-0.0122890580421644,0.159968340300288,
3.78840842784543));
#28986=CARTESIAN_POINT('Ctrl Pts',(0.127748871668302,0.0970624367746977,
3.78046874776856));
#28987=CARTESIAN_POINT('Ctrl Pts',(0.150822838766923,-0.0547116272036868,
3.77252906769167));
#28988=CARTESIAN_POINT('Ctrl Pts',(0.0358068435549273,-0.156392969151285,
3.7645893876148));
#28989=CARTESIAN_POINT('Ctrl Pts',(-0.111993083570565,-0.114884464038922,
3.75664970753792));
#28990=CARTESIAN_POINT('Ctrl Pts',(-0.157254689471112,0.0318096445201475,
3.74871002746105));
#28991=CARTESIAN_POINT('Ctrl Pts',(-0.0585374767790549,0.149379565729933,
3.74077034738417));
#28992=CARTESIAN_POINT('Ctrl Pts',(0.0937753188391016,0.130180952606797,
3.7328306673073));
#28993=CARTESIAN_POINT('Ctrl Pts',(0.160229564451327,-0.00820838113787044,
3.72489098723042));
#28994=CARTESIAN_POINT('Ctrl Pts',(0.0799812635707716,-0.139082307730405,
3.71695130715355));
#28995=CARTESIAN_POINT('Ctrl Pts',(-0.0734960639111485,-0.142615635303926,
3.70901162707667));
#28996=CARTESIAN_POINT('Ctrl Pts',(-0.15968206616318,-0.015573329490413,
3.7010719469998));
#28997=CARTESIAN_POINT('Ctrl Pts',(-0.0996667989077476,0.125727562793709,
3.69313226692292));
#28998=CARTESIAN_POINT('Ctrl Pts',(0.0516011235647474,0.151915156845068,
3.68519258684604));
#28999=CARTESIAN_POINT('Ctrl Pts',(0.155624230421734,0.039012687134034,
3.67725290676917));
#29000=CARTESIAN_POINT('Ctrl Pts',(0.117161329921862,-0.109608912278647,
3.66931322669229));
#29001=CARTESIAN_POINT('Ctrl Pts',(-0.0285718206606646,-0.157875082931424,
3.66137354661541));
#29002=CARTESIAN_POINT('Ctrl Pts',(-0.148145261817129,-0.0615944179514364,
3.65343386653854));
#29003=CARTESIAN_POINT('Ctrl Pts',(-0.132080269227278,0.0910806979574378,
3.64549418646166));
#29004=CARTESIAN_POINT('Ctrl Pts',(0.00491441507287188,0.160364393256412,
3.63755450638479));
#29005=CARTESIAN_POINT('Ctrl Pts',(0.137409572720802,0.08282210411744,3.62961482630791));
#29006=CARTESIAN_POINT('Ctrl Pts',(0.144095649384483,-0.0705502367355182,
3.62167514623104));
#29007=CARTESIAN_POINT('Ctrl Pts',(0.0188510256337537,-0.159328353333054,
3.61373546615416));
#29008=CARTESIAN_POINT('Ctrl Pts',(-0.12365316908484,-0.102229113178448,
3.60579578607729));
#29009=CARTESIAN_POINT('Ctrl Pts',(-0.152943332461211,0.0484688986126864,
3.5978561060004));
#29010=CARTESIAN_POINT('Ctrl Pts',(-0.0422020594748354,0.15478965501967,
3.58991642592354));
#29011=CARTESIAN_POINT('Ctrl Pts',(0.107178463180333,0.119388978607241,
3.58197674584666));
#29012=CARTESIAN_POINT('Ctrl Pts',(0.15842881484584,-0.0253224231037578,
3.57403706576978));
#29013=CARTESIAN_POINT('Ctrl Pts',(0.0646253585702682,-0.146847451071376,
3.56609738569291));
#29014=CARTESIAN_POINT('Ctrl Pts',(-0.0883476324694729,-0.133925685839263,
3.55815770561603));
#29015=CARTESIAN_POINT('Ctrl Pts',(-0.160431489631001,0.00162201932547174,
3.55021802553915));
#29016=CARTESIAN_POINT('Ctrl Pts',(-0.0856280199974695,0.135671703905846,
3.54227834546228));
#29017=CARTESIAN_POINT('Ctrl Pts',(0.067574708591012,0.145528716359985,
3.5343386653854));
#29018=CARTESIAN_POINT('Ctrl Pts',(0.15890720230823,0.0220936293617927,
3.52639898530853));
#29019=CARTESIAN_POINT('Ctrl Pts',(0.104748550086015,-0.121473483470044,
3.51845930523165));
#29020=CARTESIAN_POINT('Ctrl Pts',(-0.0453163640766394,-0.154011764793424,
3.51051962515478));
#29021=CARTESIAN_POINT('Ctrl Pts',(-0.153893675382528,-0.0451562300861186,
3.5025799450779));
#29022=CARTESIAN_POINT('Ctrl Pts',(-0.132305068112328,0.0543753790239735,
3.49728682502665));
#29023=CARTESIAN_POINT('Ctrl Pts',(-0.102845629995675,0.0885794229410565,
3.49464026500102));
#29024=CARTESIAN_POINT('Ctrl Pts',(-0.0326585063531114,-0.122159831625554,
4.01607920499693));
#29025=CARTESIAN_POINT('Ctrl Pts',(-0.0732860006472263,-0.111298378536929,
4.0134326449713));
#29026=CARTESIAN_POINT('Ctrl Pts',(-0.142146941432609,-0.046026227862863,
4.00813952492006));
#29027=CARTESIAN_POINT('Ctrl Pts',(-0.11572023141111,0.0947476923899126,
4.00019984484318));
#29028=CARTESIAN_POINT('Ctrl Pts',(0.0168566022920696,0.148475532407486,
3.9922601647663));
#29029=CARTESIAN_POINT('Ctrl Pts',(0.133899758227606,0.0664079633497781,
3.98432048468943));
#29030=CARTESIAN_POINT('Ctrl Pts',(0.128398460752025,-0.076535065655625,
3.97638080461255));
#29031=CARTESIAN_POINT('Ctrl Pts',(0.00531228231285306,-0.149366566296356,
3.96844112453568));
#29032=CARTESIAN_POINT('Ctrl Pts',(-0.12262429744638,-0.0854607724530698,
3.9605014444588));
#29033=CARTESIAN_POINT('Ctrl Pts',(-0.1382957240796,0.0567008670107902,
3.95256176438192));
#29034=CARTESIAN_POINT('Ctrl Pts',(-0.0273432128090029,0.146943407785525,
3.94462208430505));
#29035=CARTESIAN_POINT('Ctrl Pts',(0.108642320896687,0.102650504162914,
3.93668240422817));
#29036=CARTESIAN_POINT('Ctrl Pts',(0.145158338364007,-0.0356281987660663,
3.9287427241513));
#29037=CARTESIAN_POINT('Ctrl Pts',(0.0487702085748674,-0.141285850885848,
3.92080304407442));
#29038=CARTESIAN_POINT('Ctrl Pts',(-0.0922705732672884,-0.117585739336083,
3.91286336399754));
#29039=CARTESIAN_POINT('Ctrl Pts',(-0.148830639984962,0.0137733808691391,
3.90492368392067));
#29040=CARTESIAN_POINT('Ctrl Pts',(-0.0691246927616998,0.132521815008853,
3.89698400384379));
#29041=CARTESIAN_POINT('Ctrl Pts',(0.0738702190981043,0.129936335085374,
3.88904432376692));
#29042=CARTESIAN_POINT('Ctrl Pts',(0.149231254418321,0.00838407672456824,
3.88110464369004));
#29043=CARTESIAN_POINT('Ctrl Pts',(0.0879595373313327,-0.120844439356652,
3.87316496361317));
#29044=CARTESIAN_POINT('Ctrl Pts',(-0.0538459280560888,-0.139430540397488,
3.86522528353628));
#29045=CARTESIAN_POINT('Ctrl Pts',(-0.146351288109975,-0.0303572052832036,
3.85728560345941));
#29046=CARTESIAN_POINT('Ctrl Pts',(-0.104860734827282,0.106510495180087,
3.84934592338253));
#29047=CARTESIAN_POINT('Ctrl Pts',(0.0326379227320163,0.145859608554342,
3.84140624330567));
#29048=CARTESIAN_POINT('Ctrl Pts',(0.140254040541868,0.0516629799285589,
3.83346656322878));
#29049=CARTESIAN_POINT('Ctrl Pts',(0.119456747265108,-0.0898350983716749,
3.82552688315191));
#29050=CARTESIAN_POINT('Ctrl Pts',(-0.0107124279541533,-0.14908220306158,
3.81758720307504));
#29051=CARTESIAN_POINT('Ctrl Pts',(-0.131073547719428,-0.0718330318604663,
3.80964752299816));
#29052=CARTESIAN_POINT('Ctrl Pts',(-0.131426707047127,0.0711848302031395,
3.80170784292129));
#29053=CARTESIAN_POINT('Ctrl Pts',(-0.0114485613170311,0.149027480090653,
3.7937681628444));
#29054=CARTESIAN_POINT('Ctrl Pts',(0.119011626884504,0.0904239572457801,
3.78582848276753));
#29055=CARTESIAN_POINT('Ctrl Pts',(0.140507475162653,-0.0509696851171873,
3.77788880269065));
#29056=CARTESIAN_POINT('Ctrl Pts',(0.0333578735328136,-0.145696642552897,
3.76994912261378));
#29057=CARTESIAN_POINT('Ctrl Pts',(-0.104333438734023,-0.10702706638793,
3.7620094425369));
#29058=CARTESIAN_POINT('Ctrl Pts',(-0.146499426451047,0.0296340585675785,
3.75406976246003));
#29059=CARTESIAN_POINT('Ctrl Pts',(-0.0545338698824522,0.139162913211322,
3.74613008238315));
#29060=CARTESIAN_POINT('Ctrl Pts',(0.0873616581572035,0.121277368299088,
3.73819040230628));
#29061=CARTESIAN_POINT('Ctrl Pts',(0.149270838100714,-0.00764697786014525,
3.7302507222294));
#29062=CARTESIAN_POINT('Ctrl Pts',(0.0745110322582815,-0.129569924944816,
3.72231104215252));
#29063=CARTESIAN_POINT('Ctrl Pts',(-0.0684693807580898,-0.132861594431592,
3.71437136207565));
#29064=CARTESIAN_POINT('Ctrl Pts',(-0.148760785361007,-0.0145082086006585,
3.70643168199877));
#29065=CARTESIAN_POINT('Ctrl Pts',(-0.0928501968704667,0.117128563226408,
3.6984920019219));
#29066=CARTESIAN_POINT('Ctrl Pts',(0.0480719209830229,0.141525085336877,
3.69055232184502));
#29067=CARTESIAN_POINT('Ctrl Pts',(0.144980480870543,0.0363444569358934,
3.68261264176815));
#29068=CARTESIAN_POINT('Ctrl Pts',(0.10914820851144,-0.102112330237978,
3.67467296169127));
#29069=CARTESIAN_POINT('Ctrl Pts',(-0.0266176821405283,-0.147077388777102,
3.66673328161439));
#29070=CARTESIAN_POINT('Ctrl Pts',(-0.138013028168781,-0.0573817348965553,
3.65879360153751));
#29071=CARTESIAN_POINT('Ctrl Pts',(-0.123046783230275,0.0848513329325982,
3.65085392146064));
#29072=CARTESIAN_POINT('Ctrl Pts',(0.00457829901250977,0.149396445436689,
3.64291424138376));
#29073=CARTESIAN_POINT('Ctrl Pts',(0.128011594822289,0.0771575766133371,
3.63497456130689));
#29074=CARTESIAN_POINT('Ctrl Pts',(0.134240384562878,-0.0657250302200856,
3.62703488123001));
#29075=CARTESIAN_POINT('Ctrl Pts',(0.0175617302901878,-0.148431264334219,
3.61909520115314));
#29076=CARTESIAN_POINT('Ctrl Pts',(-0.115196045413394,-0.0952372644505018,
3.61115552107626));
#29077=CARTESIAN_POINT('Ctrl Pts',(-0.14248294000285,0.0451539211412638,
3.60321584099938));
#29078=CARTESIAN_POINT('Ctrl Pts',(-0.039315695633052,0.144202985343104,
3.59527616092251));
#29079=CARTESIAN_POINT('Ctrl Pts',(0.0998481090556468,0.111223499593951,
3.58733648084563));
#29080=CARTESIAN_POINT('Ctrl Pts',(0.147593248801005,-0.0235905235864699,
3.57939680076876));
#29081=CARTESIAN_POINT('Ctrl Pts',(0.0602053776366188,-0.136803979773886,
3.57145712069188));
#29082=CARTESIAN_POINT('Ctrl Pts',(-0.0823051924786211,-0.124765984585276,
3.56351744061501));
#29083=CARTESIAN_POINT('Ctrl Pts',(-0.149458952827898,0.00151108308231263,
3.55557776053813));
#29084=CARTESIAN_POINT('Ctrl Pts',(-0.0797715849362477,0.126392585650007,
3.54763808046126));
#29085=CARTESIAN_POINT('Ctrl Pts',(0.0629530100785864,0.135575438485168,
3.53969840038438));
#29086=CARTESIAN_POINT('Ctrl Pts',(0.148038917474527,0.020582559671896,
3.5317587203075));
#29087=CARTESIAN_POINT('Ctrl Pts',(0.097584387217902,-0.113165437019551,
3.52381904023062));
#29088=CARTESIAN_POINT('Ctrl Pts',(-0.0422170007673702,-0.143478298070691,
3.51587936015375));
#29089=CARTESIAN_POINT('Ctrl Pts',(-0.143368285256292,-0.0420678189665254,
3.50793968007687));
#29090=CARTESIAN_POINT('Ctrl Pts',(-0.123256207240696,0.0506564342650893,
3.50264656002563));
#29091=CARTESIAN_POINT('Ctrl Pts',(-0.0958116152722475,0.0825211298936389,
3.5));
#29092=CARTESIAN_POINT('Ctrl Pts',(-0.126283770505697,7.06948412972308E-5,
3.95565803263806));
#29093=CARTESIAN_POINT('Ctrl Pts',(-0.126367959766412,0.0165211867142232,
3.95462594321935));
#29094=CARTESIAN_POINT('Ctrl Pts',(-0.123384590961307,0.0329424219101817,
3.95359385380063));
#29095=CARTESIAN_POINT('Ctrl Pts',(-0.117191734428964,0.0480476838959361,
3.95256176438192));
#29096=CARTESIAN_POINT('Ctrl Pts',(-0.101311553656068,0.086781713935702,
3.9499152043563));
#29097=CARTESIAN_POINT('Ctrl Pts',(-0.0643273832325353,0.116862560860614,
3.94726864433067));
#29098=CARTESIAN_POINT('Ctrl Pts',(-0.0231710424031541,0.124520833719301,
3.94462208430505));
#29099=CARTESIAN_POINT('Ctrl Pts',(0.0179852984262271,0.132179106577988,
3.94197552427942));
#29100=CARTESIAN_POINT('Ctrl Pts',(0.0633138096614572,0.117414805370451,
3.9393289642538));
#29101=CARTESIAN_POINT('Ctrl Pts',(0.0920640681902922,0.0869862042785193,
3.93668240422817));
#29102=CARTESIAN_POINT('Ctrl Pts',(0.120814326719127,0.0565576031865874,
3.93403584420254));
#29103=CARTESIAN_POINT('Ctrl Pts',(0.132986332541567,0.0104647022102606,
3.93138928417692));
#29104=CARTESIAN_POINT('Ctrl Pts',(0.123007647154597,-0.0301913569645331,
3.9287427241513));
#29105=CARTESIAN_POINT('Ctrl Pts',(0.113028961767627,-0.0708474161393267,
3.92609616412567));
#29106=CARTESIAN_POINT('Ctrl Pts',(0.0808995851712473,-0.106066633512587,
3.92344960410005));
#29107=CARTESIAN_POINT('Ctrl Pts',(0.0413280998993647,-0.11972622360759,
3.92080304407442));
#29108=CARTESIAN_POINT('Ctrl Pts',(0.00175661462748208,-0.133385813702593,
3.91815648404879));
#29109=CARTESIAN_POINT('Ctrl Pts',(-0.0452569793199031,-0.125485776519338,
3.91550992402317));
#29110=CARTESIAN_POINT('Ctrl Pts',(-0.0781904540798746,-0.0996425712268402,
3.91286336399754));
#29111=CARTESIAN_POINT('Ctrl Pts',(-0.10807787979064,-0.0761896290779491,
3.91046158687771));
#29112=CARTESIAN_POINT('Ctrl Pts',(-0.126369304595299,-0.037959184630699,
3.90805980975789));
#29113=CARTESIAN_POINT('Ctrl Pts',(-0.126614009842867,6.71750503076223E-5,
3.90565803263806));
#29114=CARTESIAN_POINT('Ctrl Pts',(-0.0398513841857263,-0.149064942821851,
4.));
#29115=CARTESIAN_POINT('Ctrl Pts',(-0.0498814023543805,-0.14540001546545,
4.));
#29116=CARTESIAN_POINT('Ctrl Pts',(-0.0594354697797451,-0.140634945951871,
4.));
#29117=CARTESIAN_POINT('Ctrl Pts',(-0.0684028880593604,-0.13492060142061,
4.));
#29118=CARTESIAN_POINT('Ctrl Pts',(-0.0752795449518356,-0.130538561296954,
4.));
#29119=CARTESIAN_POINT('Ctrl Pts',(-0.0818109545260972,-0.125596962852027,
4.));
#29120=CARTESIAN_POINT('Ctrl Pts',(-0.0879325986341956,-0.120150358192012,
4.));
#29121=CARTESIAN_POINT('Ctrl Pts',(-0.0903223739843738,-0.118024105615282,
4.));
#29122=CARTESIAN_POINT('Ctrl Pts',(-0.0926479810229214,-0.115821878910758,
4.));
#29123=CARTESIAN_POINT('Ctrl Pts',(-0.0948977224364798,-0.11355536832373,
4.));
#29124=CARTESIAN_POINT('Ctrl Pts',(-0.1022475948872,-0.106150711227375,
4.));
#29125=CARTESIAN_POINT('Ctrl Pts',(-0.108817076574654,-0.0980392058992304,
4.));
#29126=CARTESIAN_POINT('Ctrl Pts',(-0.114476228961537,-0.0893439955398699,
4.));
#29127=CARTESIAN_POINT('Ctrl Pts',(-0.117310911144628,-0.0849885450768213,
4.));
#29128=CARTESIAN_POINT('Ctrl Pts',(-0.119916487835761,-0.0804862654238585,
4.));
#29129=CARTESIAN_POINT('Ctrl Pts',(-0.122271719969265,-0.0758513570938915,
4.));
#29130=CARTESIAN_POINT('Ctrl Pts',(-0.123706258421051,-0.073028300238791,
4.));
#29131=CARTESIAN_POINT('Ctrl Pts',(-0.12504717142243,-0.0701567413128179,
4.));
#29132=CARTESIAN_POINT('Ctrl Pts',(-0.126284991686486,-0.067251866211871,
4.));
#29133=CARTESIAN_POINT('Ctrl Pts',(-0.1295973650463,-0.0594784994498528,
4.));
#29134=CARTESIAN_POINT('Ctrl Pts',(-0.132185052379765,-0.051445045564302,
4.));
#29135=CARTESIAN_POINT('Ctrl Pts',(-0.133964990884521,-0.0432169428549209,
4.));
#29136=CARTESIAN_POINT('Ctrl Pts',(-0.135518726559135,-0.0360345055517295,
4.));
#29137=CARTESIAN_POINT('Ctrl Pts',(-0.13645631947854,-0.0287032207927444,
4.));
#29138=CARTESIAN_POINT('Ctrl Pts',(-0.136789702571871,-0.0212983790736885,
4.));
#29139=CARTESIAN_POINT('Ctrl Pts',(-0.13693233353465,-0.0181303728827948,
4.));
#29140=CARTESIAN_POINT('Ctrl Pts',(-0.136963744111631,-0.0149584576035291,
4.));
#29141=CARTESIAN_POINT('Ctrl Pts',(-0.136886254945713,-0.0117904221806244,
4.));
#29142=CARTESIAN_POINT('Ctrl Pts',(-0.136677592311597,-0.00325954423806801,
4.));
#29143=CARTESIAN_POINT('Ctrl Pts',(-0.135681410366555,0.00524856144622462,
4.));
#29144=CARTESIAN_POINT('Ctrl Pts',(-0.133925248777689,0.0136159175851835,
4.));
#29145=CARTESIAN_POINT('Ctrl Pts',(-0.132934632228228,0.018335780221422,
4.));
#29146=CARTESIAN_POINT('Ctrl Pts',(-0.131701699385377,0.0230107212566983,
4.));
#29147=CARTESIAN_POINT('Ctrl Pts',(-0.130227956640556,0.0276173752808998,
4.));
#29148=CARTESIAN_POINT('Ctrl Pts',(-0.129158656751422,0.030959813881302,
4.));
#29149=CARTESIAN_POINT('Ctrl Pts',(-0.12796229886657,0.0342658696738965,
4.));
#29150=CARTESIAN_POINT('Ctrl Pts',(-0.126644858507038,0.0375136883583919,
4.));
#29151=CARTESIAN_POINT('Ctrl Pts',(-0.124572648602295,0.042622201998594,
4.));
#29152=CARTESIAN_POINT('Ctrl Pts',(-0.122198572282107,0.0475953519381505,
4.));
#29153=CARTESIAN_POINT('Ctrl Pts',(-0.119526530046339,0.0523977893098404,
4.));
#29154=CARTESIAN_POINT('Ctrl Pts',(-0.116935312520942,0.0570549611597328,
4.));
#29155=CARTESIAN_POINT('Ctrl Pts',(-0.11406058633243,0.0615550019486321,
4.));
#29156=CARTESIAN_POINT('Ctrl Pts',(-0.11092106856286,0.0658392337664117,
4.));
#29157=CARTESIAN_POINT('Ctrl Pts',(-0.10710607669906,0.071045227402084,
4.));
#29158=CARTESIAN_POINT('Ctrl Pts',(-0.102897192277319,0.075940267594365,
4.));
#29159=CARTESIAN_POINT('Ctrl Pts',(-0.0982968852906839,0.0804596595786888,
4.));
#29160=CARTESIAN_POINT('Ctrl Pts',(-0.0975398380300018,0.0812033911017416,
4.));
#29161=CARTESIAN_POINT('Ctrl Pts',(-0.0967721750025885,0.0819369232370377,
4.));
#29162=CARTESIAN_POINT('Ctrl Pts',(-0.0959941513168557,0.0826601513985347,
4.));
#29163=CARTESIAN_POINT('Origin',(0.,0.,3.7));
#29164=CARTESIAN_POINT('Origin',(0.,0.,3.4));
#29165=CARTESIAN_POINT('Origin',(1.,0.,3.8));
#29166=CARTESIAN_POINT('',(0.8,2.44929359829471E-17,4.));
#29167=CARTESIAN_POINT('Origin',(1.,0.,4.));
#29168=CARTESIAN_POINT('',(0.8,2.44929359829471E-17,3.6));
#29169=CARTESIAN_POINT('',(0.8,2.44929359829471E-17,3.8));
#29170=CARTESIAN_POINT('Origin',(1.,0.,3.6));
#29171=CARTESIAN_POINT('Origin',(1.4,-0.6,3.6));
#29172=CARTESIAN_POINT('',(1.4,-0.6,3.6));
#29173=CARTESIAN_POINT('',(1.4,0.6,3.6));
#29174=CARTESIAN_POINT('',(1.4,-0.6,3.6));
#29175=CARTESIAN_POINT('',(1.4,0.6,4.));
#29176=CARTESIAN_POINT('',(1.4,0.6,3.6));
#29177=CARTESIAN_POINT('',(1.4,-0.6,4.));
#29178=CARTESIAN_POINT('',(1.4,-0.6,4.));
#29179=CARTESIAN_POINT('',(1.4,-0.6,3.6));
#29180=CARTESIAN_POINT('Origin',(0.7,0.,3.6));
#29181=CARTESIAN_POINT('',(0.4,0.6,3.6));
#29182=CARTESIAN_POINT('',(0.4,-0.6,3.6));
#29183=CARTESIAN_POINT('',(0.4,-0.3,3.6));
#29184=CARTESIAN_POINT('',(1.4,0.6,3.6));
#29185=CARTESIAN_POINT('',(0.,-0.6,3.6));
#29186=CARTESIAN_POINT('Origin',(0.4,0.6,2.6));
#29187=CARTESIAN_POINT('',(-0.4,0.6,4.));
#29188=CARTESIAN_POINT('',(0.4,0.6,4.));
#29189=CARTESIAN_POINT('',(0.4,0.6,2.6));
#29190=CARTESIAN_POINT('',(0.4,0.6,2.6));
#29191=CARTESIAN_POINT('',(-0.4,0.6,2.6));
#29192=CARTESIAN_POINT('',(0.4,0.6,2.6));
#29193=CARTESIAN_POINT('',(-0.4,0.6,2.6));
#29194=CARTESIAN_POINT('Origin',(0.4,-0.6,2.6));
#29195=CARTESIAN_POINT('',(0.4,-0.6,2.6));
#29196=CARTESIAN_POINT('',(0.4,-0.6,2.6));
#29197=CARTESIAN_POINT('',(0.4,-0.6,2.6));
#29198=CARTESIAN_POINT('Origin',(-0.4,-0.6,2.6));
#29199=CARTESIAN_POINT('',(-0.4,-0.6,4.));
#29200=CARTESIAN_POINT('',(-0.4,-0.6,4.));
#29201=CARTESIAN_POINT('',(-0.4,-0.6,2.6));
#29202=CARTESIAN_POINT('',(-0.4,-0.6,2.6));
#29203=CARTESIAN_POINT('',(-0.4,-0.6,2.6));
#29204=CARTESIAN_POINT('Origin',(-0.4,0.6,2.6));
#29205=CARTESIAN_POINT('',(-0.4,0.6,2.6));
#29206=CARTESIAN_POINT('',(-0.4,0.6,4.));
#29207=CARTESIAN_POINT('Origin',(0.,0.,4.));
#29208=CARTESIAN_POINT('Origin',(0.,0.,2.6));
#36453=UNCERTAINTY_MEASURE_WITH_UNIT(LENGTH_MEASURE(0.001),#36483,
'DISTANCE_ACCURACY_VALUE',
'Maximum model space distance between geometric entities at asserted c
onnectivities');
#36463=UNCERTAINTY_MEASURE_WITH_UNIT(LENGTH_MEASURE(0.001),#36483,
'DISTANCE_ACCURACY_VALUE',
'Maximum model space distance between geometric entities at asserted c
onnectivities');
#36472=(
GEOMETRIC_REPRESENTATION_CONTEXT(3)
GLOBAL_UNCERTAINTY_ASSIGNED_CONTEXT((#36453))
GLOBAL_UNIT_ASSIGNED_CONTEXT((#36483,#36485,#36486))
REPRESENTATION_CONTEXT('','3D')
);
#36482=(
GEOMETRIC_REPRESENTATION_CONTEXT(3)
GLOBAL_UNCERTAINTY_ASSIGNED_CONTEXT((#36463))
GLOBAL_UNIT_ASSIGNED_CONTEXT((#36483,#36485,#36486))
REPRESENTATION_CONTEXT('','3D')
);
#36483=(
LENGTH_UNIT()
NAMED_UNIT(*)
SI_UNIT(.CENTI.,.METRE.)
);
#36485=(
NAMED_UNIT(*)
PLANE_ANGLE_UNIT()
SI_UNIT($,.RADIAN.)
);
#36486=(
NAMED_UNIT(*)
SI_UNIT($,.STERADIAN.)
SOLID_ANGLE_UNIT()
);
#36495=SHAPE_DEFINITION_REPRESENTATION(#36513,#36562);
#36513=PRODUCT_DEFINITION_SHAPE('',$,#36581);
#36562=SHAPE_REPRESENTATION('',(#10401),#36472);
#36572=PRODUCT_DEFINITION_CONTEXT('part definition',#36628,'design');
#36581=PRODUCT_DEFINITION('Fixed contact terminal',
'Fixed contact terminal',#36599,#36572);
#36599=PRODUCT_DEFINITION_FORMATION('',$,#36638);
#36628=APPLICATION_CONTEXT(
'Core Data for Automotive Mechanical Design Process');
#36629=PRODUCT_CONTEXT('part definition',#36628,'mechanical');
#36638=PRODUCT('Fixed contact terminal','Fixed contact terminal',$,(#36629));
#36653=PRESENTATION_STYLE_ASSIGNMENT((#36667));
#36667=SURFACE_STYLE_USAGE(.BOTH.,#36681);
#36681=SURFACE_SIDE_STYLE('',(#36695));
#36695=SURFACE_STYLE_FILL_AREA(#36709);
#36709=FILL_AREA_STYLE('Contact gray',(#36723));
#36723=FILL_AREA_STYLE_COLOUR('Contact gray',#36737);
#36737=COLOUR_RGB('Contact gray',0.725490196078431,0.752941176470588,0.792156862745098);
ENDSEC;
END-ISO-10303-21;
